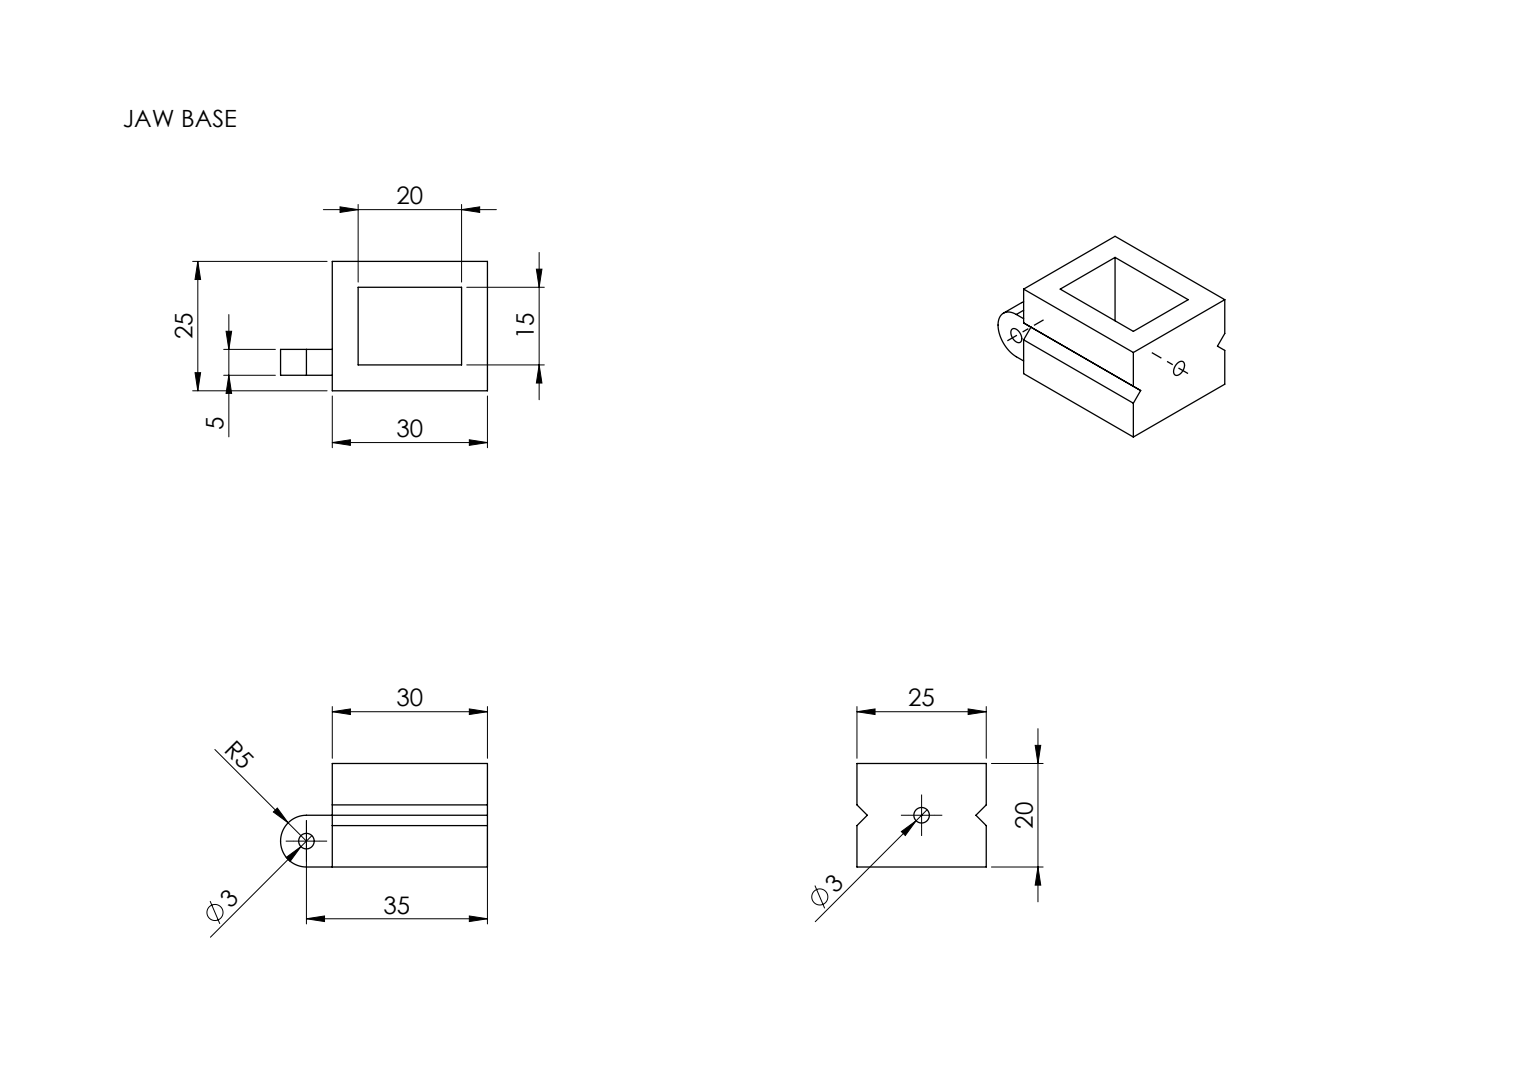
ISO-10303-21;
HEADER;
FILE_DESCRIPTION (('STEP AP214'),
    '1' );
FILE_NAME ('jaw base.step',
    '2026-10-04T07:56:41',
    ( '' ),
    ( '' ),
    'SwSTEP 2.0',
    'SolidWorks 2026',
    '' );
FILE_SCHEMA (( 'AUTOMOTIVE_DESIGN' ));
ENDSEC;

DATA;
#2=DIRECTION ( 'NONE',  ( -0.000000000000000000, 2.775557561562891351E-16, -1.000000000000000000 ) ) ;
#9=VERTEX_POINT ( 'NONE', #7435 ) ;
#11=DIRECTION ( 'NONE',  ( 0.000000000000000000, -1.000000000000000000, 0.000000000000000000 ) ) ;
#43=EDGE_CURVE ( 'NONE', #1966, #5555, #3595, .T. ) ;
#44=LINE ( 'NONE', #810, #6447 ) ;
#74=CARTESIAN_POINT ( 'NONE',  ( 54.99999999999999289, 1.301042606982605715E-15, -7.500000000000002665 ) ) ;
#76=EDGE_LOOP ( 'NONE', ( #356, #276, #5543, #6009 ) ) ;
#88=FACE_OUTER_BOUND ( 'NONE', #2763, .T. ) ;
#100=CARTESIAN_POINT ( 'NONE',  ( 50.00000000000000000, -1.734723475976807094E-15, 12.50000000000000000 ) ) ;
#116=DIRECTION ( 'NONE',  ( 0.000000000000000000, 0.000000000000000000, 1.000000000000000000 ) ) ;
#129=AXIS2_PLACEMENT_3D ( 'NONE', #1955, #4587, #1439 ) ;
#148=LINE ( 'NONE', #5288, #6329 ) ;
#154=LINE ( 'NONE', #7878, #4231 ) ;
#158=EDGE_CURVE ( 'NONE', #4876, #5889, #5061, .T. ) ;
#177=LINE ( 'NONE', #1487, #3670 ) ;
#187=VECTOR ( 'NONE', #1383, 1000.000000000000000 ) ;
#189=AXIS2_PLACEMENT_3D ( 'NONE', #3637, #5920, #5243 ) ;
#192=FACE_OUTER_BOUND ( 'NONE', #662, .T. ) ;
#210=VERTEX_POINT ( 'NONE', #510 ) ;
#226=EDGE_CURVE ( 'NONE', #6118, #4574, #2581, .T. ) ;
#266=CARTESIAN_POINT ( 'NONE',  ( 54.99999999999999289, -1.301042606982604729E-15, 7.499999999999997335 ) ) ;
#271=CIRCLE ( 'NONE', #522, 5.000000000000000888 ) ;
#276=ORIENTED_EDGE ( 'NONE', *, *, #1868, .F. ) ;
#280=EDGE_CURVE ( 'NONE', #6915, #2088, #1958, .T. ) ;
#291=ADVANCED_FACE ( 'NONE', ( #7854, #719 ), #1914, .F. ) ;
#295=CARTESIAN_POINT ( 'NONE',  ( 54.99999999999999289, 1.301042606982605715E-15, -7.500000000000002665 ) ) ;
#299=CARTESIAN_POINT ( 'NONE',  ( 50.00000000000000000, 1.734723475976807094E-15, -12.50000000000000000 ) ) ;
#305=CARTESIAN_POINT ( 'NONE',  ( 54.99999999999999289, -9.999999999999994671, -1.500000000000000666 ) ) ;
#314=CARTESIAN_POINT ( 'NONE',  ( 45.00000000000000000, -14.99999999999999467, 4.499999999999999112 ) ) ;
#328=EDGE_CURVE ( 'NONE', #3916, #5740, #1998, .T. ) ;
#344=CARTESIAN_POINT ( 'NONE',  ( 80.00000000000000000, -9.999999999999991118, -10.50000000000000888 ) ) ;
#348=VERTEX_POINT ( 'NONE', #4548 ) ;
#352=FACE_OUTER_BOUND ( 'NONE', #3772, .T. ) ;
#356=ORIENTED_EDGE ( 'NONE', *, *, #5085, .F. ) ;
#359=EDGE_CURVE ( 'NONE', #1450, #210, #2081, .T. ) ;
#373=CARTESIAN_POINT ( 'NONE',  ( 75.00000000000000000, -19.99999999999999645, -7.500000000000006217 ) ) ;
#397=AXIS2_PLACEMENT_3D ( 'NONE', #4050, #2120, #1311 ) ;
#414=EDGE_CURVE ( 'NONE', #7949, #1490, #44, .T. ) ;
#424=FACE_OUTER_BOUND ( 'NONE', #5365, .T. ) ;
#440=ORIENTED_EDGE ( 'NONE', *, *, #4555, .F. ) ;
#443=CARTESIAN_POINT ( 'NONE',  ( 50.00000000000000000, -9.999999999999994671, -1.500000000000000666 ) ) ;
#463=CARTESIAN_POINT ( 'NONE',  ( 54.99999999999999289, -19.99999999999999645, -12.50000000000000355 ) ) ;
#476=LINE ( 'NONE', #8193, #724 ) ;
#477=ADVANCED_FACE ( 'NONE', ( #88 ), #7132, .F. ) ;
#481=PLANE ( 'NONE',  #6922 ) ;
#482=ORIENTED_EDGE ( 'NONE', *, *, #2370, .T. ) ;
#499=VECTOR ( 'NONE', #7220, 1000.000000000000000 ) ;
#510=CARTESIAN_POINT ( 'NONE',  ( 50.00000000000000000, -12.00000000000000711, 12.49999999999999822 ) ) ;
#514=CARTESIAN_POINT ( 'NONE',  ( 80.00000000000000000, -7.999999999999992895, -12.50000000000000178 ) ) ;
#518=SURFACE_STYLE_USAGE ( .BOTH. , #4233 ) ;
#519=ORIENTED_EDGE ( 'NONE', *, *, #6332, .T. ) ;
#522=AXIS2_PLACEMENT_3D ( 'NONE', #3905, #2648, #1459 ) ;
#523=DIRECTION ( 'NONE',  ( 1.000000000000000000, 0.000000000000000000, 0.000000000000000000 ) ) ;
#548=PLANE ( 'NONE',  #3363 ) ;
#561=ORIENTED_EDGE ( 'NONE', *, *, #611, .F. ) ;
#562=LINE ( 'NONE', #3139, #7733 ) ;
#585=VECTOR ( 'NONE', #4039, 1000.000000000000000 ) ;
#589=AXIS2_PLACEMENT_3D ( 'NONE', #100, #733, #2054 ) ;
#611=EDGE_CURVE ( 'NONE', #5740, #6524, #3988, .T. ) ;
#618=FACE_OUTER_BOUND ( 'NONE', #620, .T. ) ;
#620=EDGE_LOOP ( 'NONE', ( #5338, #2831, #6955, #4736 ) ) ;
#637=AXIS2_PLACEMENT_3D ( 'NONE', #2916, #7427, #1567 ) ;
#641=ORIENTED_EDGE ( 'NONE', *, *, #1752, .T. ) ;
#662=EDGE_LOOP ( 'NONE', ( #2589, #4451, #6768, #2881 ) ) ;
#675=CARTESIAN_POINT ( 'NONE',  ( 50.00000000000000000, -20.00000000000000355, 12.49999999999999645 ) ) ;
#678=CARTESIAN_POINT ( 'NONE',  ( 40.00000000000000000, -9.999999999999991118, 9.499999999999998224 ) ) ;
#694=EDGE_CURVE ( 'NONE', #3832, #7792, #3206, .T. ) ;
#700=AXIS2_PLACEMENT_3D ( 'NONE', #5107, #2634, #5148 ) ;
#703=DIRECTION ( 'NONE',  ( -1.000000000000000000, -0.000000000000000000, -0.000000000000000000 ) ) ;
#719=FACE_OUTER_BOUND ( 'NONE', #1634, .T. ) ;
#722=FACE_BOUND ( 'NONE', #2870, .T. ) ;
#724=VECTOR ( 'NONE', #4868, 1000.000000000000114 ) ;
#733=DIRECTION ( 'NONE',  ( 0.000000000000000000, -2.168404344971010347E-16, 1.000000000000000000 ) ) ;
#734=EDGE_CURVE ( 'NONE', #4784, #5781, #271, .T. ) ;
#740=DIRECTION ( 'NONE',  ( 0.000000000000000000, 0.000000000000000000, -1.000000000000000000 ) ) ;
#748=LINE ( 'NONE', #5933, #187 ) ;
#758=CARTESIAN_POINT ( 'NONE',  ( 45.00000000000000000, -15.00000000000000000, -4.163336342344337027E-15 ) ) ;
#778=DIRECTION ( 'NONE',  ( -0.000000000000000000, 1.000000000000000000, 1.734723475976807094E-16 ) ) ;
#781=DIRECTION ( 'NONE',  ( -0.000000000000000000, -1.387778780781445676E-16, 1.000000000000000000 ) ) ;
#784=DIRECTION ( 'NONE',  ( 1.000000000000000000, 0.000000000000000000, 0.000000000000000000 ) ) ;
#789=ORIENTED_EDGE ( 'NONE', *, *, #1868, .T. ) ;
#791=LINE ( 'NONE', #5465, #585 ) ;
#802=VECTOR ( 'NONE', #5944, 1000.000000000000000 ) ;
#810=CARTESIAN_POINT ( 'NONE',  ( 50.00000000000000000, -19.99999999999999645, -12.50000000000000355 ) ) ;
#832=ORIENTED_EDGE ( 'NONE', *, *, #1520, .T. ) ;
#842=EDGE_CURVE ( 'NONE', #7792, #3832, #1325, .T. ) ;
#845=FACE_OUTER_BOUND ( 'NONE', #4405, .T. ) ;
#852=CYLINDRICAL_SURFACE ( 'NONE', #6905, 1.500000000000000666 ) ;
#858=ORIENTED_EDGE ( 'NONE', *, *, #2230, .T. ) ;
#867=DIRECTION ( 'NONE',  ( 0.000000000000000000, -1.000000000000000000, 3.469446951953615175E-16 ) ) ;
#871=CARTESIAN_POINT ( 'NONE',  ( 50.00000000000000000, -9.999999999999992895, 4.499999999999999112 ) ) ;
#876=CARTESIAN_POINT ( 'NONE',  ( 50.00000000000000000, -12.00000000000000355, -12.50000000000000178 ) ) ;
#879=ADVANCED_FACE ( 'NONE', ( #1961 ), #7726, .F. ) ;
#889=FACE_BOUND ( 'NONE', #8067, .T. ) ;
#893=CARTESIAN_POINT ( 'NONE',  ( 50.00000000000000000, -9.999999999999994671, 10.50000000000000533 ) ) ;
#903=EDGE_CURVE ( 'NONE', #1902, #2390, #2584, .T. ) ;
#914=VERTEX_POINT ( 'NONE', #3261 ) ;
#918=ORIENTED_EDGE ( 'NONE', *, *, #4017, .T. ) ;
#957=PLANE ( 'NONE',  #3547 ) ;
#960=ADVANCED_FACE ( 'NONE', ( #722, #3931 ), #2758, .F. ) ;
#968=EDGE_LOOP ( 'NONE', ( #6723, #4873, #5987, #7324 ) ) ;
#992=APPLICATION_CONTEXT ( 'automotive_design' ) ;
#1003=ORIENTED_EDGE ( 'NONE', *, *, #842, .F. ) ;
#1013=DIRECTION ( 'NONE',  ( 0.000000000000000000, 0.7071067811865442421, -0.7071067811865509034 ) ) ;
#1022=DIRECTION ( 'NONE',  ( 0.000000000000000000, 0.000000000000000000, -1.000000000000000000 ) ) ;
#1040=EDGE_LOOP ( 'NONE', ( #1925, #1101, #1165, #6177 ) ) ;
#1060=EDGE_CURVE ( 'NONE', #6118, #5503, #2083, .T. ) ;
#1063=CYLINDRICAL_SURFACE ( 'NONE', #189, 1.500000000000000666 ) ;
#1072=MECHANICAL_DESIGN_GEOMETRIC_PRESENTATION_REPRESENTATION('',(#7261),#2289);
#1081=LINE ( 'NONE', #4358, #6236 ) ;
#1101=ORIENTED_EDGE ( 'NONE', *, *, #5827, .T. ) ;
#1116=ORIENTED_EDGE ( 'NONE', *, *, #8084, .T. ) ;
#1119=ORIENTED_EDGE ( 'NONE', *, *, #4522, .F. ) ;
#1122=VECTOR ( 'NONE', #1414, 1000.000000000000000 ) ;
#1133=VECTOR ( 'NONE', #778, 1000.000000000000000 ) ;
#1135=PRODUCT_DEFINITION ( 'UNKNOWN', '', #8199, #8065 ) ;
#1159=ADVANCED_FACE ( 'NONE', ( #6622 ), #6113, .F. ) ;
#1163=DIRECTION ( 'NONE',  ( 0.000000000000000000, 2.775557561562891351E-16, -1.000000000000000000 ) ) ;
#1165=ORIENTED_EDGE ( 'NONE', *, *, #4237, .T. ) ;
#1166=DIRECTION ( 'NONE',  ( 1.000000000000000000, -0.000000000000000000, -0.000000000000000000 ) ) ;
#1176=ORIENTED_EDGE ( 'NONE', *, *, #6774, .T. ) ;
#1192=CARTESIAN_POINT ( 'NONE',  ( 50.00000000000000000, -12.00000000000000355, -12.50000000000000178 ) ) ;
#1200=ORIENTED_EDGE ( 'NONE', *, *, #6332, .F. ) ;
#1203=CARTESIAN_POINT ( 'NONE',  ( 45.00000000000000000, -19.99999999999999645, -12.50000000000000355 ) ) ;
#1207=ORIENTED_EDGE ( 'NONE', *, *, #4767, .T. ) ;
#1229=EDGE_CURVE ( 'NONE', #4621, #6524, #2166, .T. ) ;
#1244=ORIENTED_EDGE ( 'NONE', *, *, #6774, .F. ) ;
#1258=CARTESIAN_POINT ( 'NONE',  ( 75.00000000000000000, -30.00000000000000000, -7.500000000000007105 ) ) ;
#1289=EDGE_CURVE ( 'NONE', #5070, #3705, #5351, .T. ) ;
#1294=CARTESIAN_POINT ( 'NONE',  ( 46.49999999999999289, -14.99999999999999467, 9.499999999999996447 ) ) ;
#1299=CARTESIAN_POINT ( 'NONE',  ( 80.00000000000000000, 1.734723475976807094E-15, -12.50000000000000000 ) ) ;
#1302=ORIENTED_EDGE ( 'NONE', *, *, #3633, .T. ) ;
#1311=DIRECTION ( 'NONE',  ( 0.000000000000000000, -1.000000000000000000, 8.673617379884033007E-17 ) ) ;
#1317=DIRECTION ( 'NONE',  ( -0.000000000000000000, 0.7071067811865484609, -0.7071067811865465735 ) ) ;
#1320=EDGE_CURVE ( 'NONE', #9, #5499, #4213, .T. ) ;
#1325=CIRCLE ( 'NONE', #4616, 1.500000000000000666 ) ;
#1328=VECTOR ( 'NONE', #5772, 1000.000000000000000 ) ;
#1348=AXIS2_PLACEMENT_3D ( 'NONE', #6049, #867, #2180 ) ;
#1353=MECHANICAL_DESIGN_GEOMETRIC_PRESENTATION_REPRESENTATION('',(#7140),#3380);
#1375=DIRECTION ( 'NONE',  ( -1.000000000000000000, -0.000000000000000000, -0.000000000000000000 ) ) ;
#1383=DIRECTION ( 'NONE',  ( -0.000000000000000000, 2.775557561562891351E-16, -1.000000000000000000 ) ) ;
#1393=LINE ( 'NONE', #3386, #802 ) ;
#1414=DIRECTION ( 'NONE',  ( -0.000000000000000000, -3.469446951953614682E-16, -1.000000000000000000 ) ) ;
#1419=DIRECTION ( 'NONE',  ( -1.000000000000000000, -0.000000000000000000, -0.000000000000000000 ) ) ;
#1421=APPLICATION_CONTEXT ( 'automotive_design' ) ;
#1439=DIRECTION ( 'NONE',  ( 0.000000000000000000, 0.000000000000000000, -1.000000000000000000 ) ) ;
#1445=LINE ( 'NONE', #2167, #3270 ) ;
#1450=VERTEX_POINT ( 'NONE', #893 ) ;
#1451=VECTOR ( 'NONE', #6786, 1000.000000000000000 ) ;
#1459=DIRECTION ( 'NONE',  ( 0.000000000000000000, 1.000000000000000000, 0.000000000000000000 ) ) ;
#1464=ADVANCED_FACE ( 'NONE', ( #7342 ), #4174, .T. ) ;
#1481=AXIS2_PLACEMENT_3D ( 'NONE', #6071, #6783, #2872 ) ;
#1487=CARTESIAN_POINT ( 'NONE',  ( 80.00000000000000000, -1.734723475976807094E-15, 12.50000000000000000 ) ) ;
#1490=VERTEX_POINT ( 'NONE', #5600 ) ;
#1499=LINE ( 'NONE', #1630, #2833 ) ;
#1507=ORIENTED_EDGE ( 'NONE', *, *, #1229, .T. ) ;
#1508=CARTESIAN_POINT ( 'NONE',  ( 80.00000000000000000, -12.00000000000000355, -12.50000000000000178 ) ) ;
#1511=ORIENTED_EDGE ( 'NONE', *, *, #6199, .T. ) ;
#1520=EDGE_CURVE ( 'NONE', #5848, #6118, #2330, .T. ) ;
#1526=DIRECTION ( 'NONE',  ( -0.000000000000000000, -8.673617379884033007E-17, -1.000000000000000000 ) ) ;
#1538=AXIS2_PLACEMENT_3D ( 'NONE', #2727, #3719, #7552 ) ;
#1539=AXIS2_PLACEMENT_3D ( 'NONE', #6210, #4308, #8076 ) ;
#1544=EDGE_LOOP ( 'NONE', ( #2817, #1646, #7710, #7360 ) ) ;
#1549=CLOSED_SHELL ( 'NONE', ( #879, #7015, #477, #7270, #2468, #1870, #1464, #4583, #5249, #6031, #2053, #5963, #7130, #6092, #5785, #960, #4435, #7621, #3038, #8204, #1159, #291, #8313, #7524, #5577, #7294, #6000 ) ) ;
#1563=DIRECTION ( 'NONE',  ( 0.000000000000000000, -1.734723475976807094E-16, 1.000000000000000000 ) ) ;
#1567=DIRECTION ( 'NONE',  ( 0.000000000000000000, 1.000000000000000000, 1.734723475976807094E-16 ) ) ;
#1574=CARTESIAN_POINT ( 'NONE',  ( 43.50000000000000711, -14.99999999999999467, 4.499999999999999112 ) ) ;
#1581=DIRECTION ( 'NONE',  ( 1.000000000000000000, 0.000000000000000000, 0.000000000000000000 ) ) ;
#1601=VECTOR ( 'NONE', #2366, 1000.000000000000000 ) ;
#1603=FACE_OUTER_BOUND ( 'NONE', #4496, .T. ) ;
#1604=VECTOR ( 'NONE', #3130, 1000.000000000000000 ) ;
#1612=DIRECTION ( 'NONE',  ( 0.000000000000000000, -1.000000000000000000, -2.168404344971010347E-16 ) ) ;
#1614=DIRECTION ( 'NONE',  ( -0.000000000000000000, -0.000000000000000000, 1.000000000000000000 ) ) ;
#1630=CARTESIAN_POINT ( 'NONE',  ( 50.00000000000000000, -9.999999999999991118, -10.50000000000000888 ) ) ;
#1632=EDGE_LOOP ( 'NONE', ( #7359, #4290, #4858, #4408, #7822, #4478, #3099, #1119, #7706, #6680, #5713, #6083, #5517, #2025 ) ) ;
#1634=EDGE_LOOP ( 'NONE', ( #8213, #7096, #1511, #918, #7592 ) ) ;
#1646=ORIENTED_EDGE ( 'NONE', *, *, #7805, .F. ) ;
#1647=CARTESIAN_POINT ( 'NONE',  ( 45.00000000000000000, -19.99999999999999645, 4.500000000000000000 ) ) ;
#1658=VERTEX_POINT ( 'NONE', #1294 ) ;
#1660=CARTESIAN_POINT ( 'NONE',  ( 50.00000000000000000, -9.999999999999994671, 1.500000000000000666 ) ) ;
#1670=SURFACE_STYLE_FILL_AREA ( #2933 ) ;
#1673=VERTEX_POINT ( 'NONE', #4445 ) ;
#1701=LINE ( 'NONE', #3757, #1884 ) ;
#1703=DIRECTION ( 'NONE',  ( -0.000000000000000000, -0.000000000000000000, 1.000000000000000000 ) ) ;
#1710=CARTESIAN_POINT ( 'NONE',  ( 54.99999999999999289, -30.00000000000000000, -7.500000000000007105 ) ) ;
#1712=( NAMED_UNIT ( * ) SI_UNIT ( $, .STERADIAN. ) SOLID_ANGLE_UNIT ( ) );
#1715=CARTESIAN_POINT ( 'NONE',  ( 75.00000000000000000, -19.99999999999999645, -12.50000000000000355 ) ) ;
#1716=PRODUCT ( 'jaw base', 'jaw base', '', ( #5739 ) ) ;
#1717=ORIENTED_EDGE ( 'NONE', *, *, #5266, .F. ) ;
#1732=LINE ( 'NONE', #8253, #1601 ) ;
#1740=( LENGTH_UNIT ( ) NAMED_UNIT ( * ) SI_UNIT ( .MILLI., .METRE. ) );
#1741=ORIENTED_EDGE ( 'NONE', *, *, #7805, .T. ) ;
#1744=VECTOR ( 'NONE', #5258, 1000.000000000000000 ) ;
#1750=DIRECTION ( 'NONE',  ( 1.000000000000000000, -0.000000000000000000, -0.000000000000000000 ) ) ;
#1752=EDGE_CURVE ( 'NONE', #3497, #6231, #2813, .T. ) ;
#1756=DIRECTION ( 'NONE',  ( 1.000000000000000000, 0.000000000000000000, 0.000000000000000000 ) ) ;
#1793=EDGE_CURVE ( 'NONE', #5848, #1966, #154, .T. ) ;
#1797=( LENGTH_UNIT ( ) NAMED_UNIT ( * ) SI_UNIT ( .MILLI., .METRE. ) );
#1804=AXIS2_PLACEMENT_3D ( 'NONE', #5339, #7884, #7325 ) ;
#1812=VECTOR ( 'NONE', #4475, 1000.000000000000000 ) ;
#1819=VERTEX_POINT ( 'NONE', #871 ) ;
#1827=ORIENTED_EDGE ( 'NONE', *, *, #6199, .F. ) ;
#1838=LINE ( 'NONE', #4470, #1924 ) ;
#1857=DIRECTION ( 'NONE',  ( 1.000000000000000000, 0.000000000000000000, 0.000000000000000000 ) ) ;
#1860=ORIENTED_EDGE ( 'NONE', *, *, #3440, .F. ) ;
#1868=EDGE_CURVE ( 'NONE', #210, #8159, #4313, .T. ) ;
#1870=ADVANCED_FACE ( 'NONE', ( #2353, #3017 ), #481, .T. ) ;
#1884=VECTOR ( 'NONE', #8224, 1000.000000000000000 ) ;
#1901=CARTESIAN_POINT ( 'NONE',  ( 50.00000000000000000, -7.999999999999992895, -12.50000000000000178 ) ) ;
#1902=VERTEX_POINT ( 'NONE', #6846 ) ;
#1910=DIRECTION ( 'NONE',  ( -0.000000000000000000, 0.7071067811865442421, 0.7071067811865509034 ) ) ;
#1914=PLANE ( 'NONE',  #6045 ) ;
#1918=LINE ( 'NONE', #514, #2199 ) ;
#1919=EDGE_CURVE ( 'NONE', #5503, #914, #7407, .T. ) ;
#1924=VECTOR ( 'NONE', #8233, 1000.000000000000000 ) ;
#1925=ORIENTED_EDGE ( 'NONE', *, *, #1060, .T. ) ;
#1955=CARTESIAN_POINT ( 'NONE',  ( 50.00000000000000000, -9.999999999999994671, 0.000000000000000000 ) ) ;
#1958=LINE ( 'NONE', #4465, #4286 ) ;
#1961=FACE_OUTER_BOUND ( 'NONE', #7933, .T. ) ;
#1966=VERTEX_POINT ( 'NONE', #6133 ) ;
#1982=ORIENTED_EDGE ( 'NONE', *, *, #7035, .T. ) ;
#1998=LINE ( 'NONE', #6413, #1328 ) ;
#2001=CARTESIAN_POINT ( 'NONE',  ( 45.00000000000000000, -14.99999999999999467, -12.50000000000000178 ) ) ;
#2002=DIRECTION ( 'NONE',  ( 1.000000000000000000, 0.000000000000000000, 0.000000000000000000 ) ) ;
#2006=ORIENTED_EDGE ( 'NONE', *, *, #158, .F. ) ;
#2025=ORIENTED_EDGE ( 'NONE', *, *, #6810, .F. ) ;
#2026=CARTESIAN_POINT ( 'NONE',  ( 45.00000000000000000, -19.99999999999999645, 9.500000000000000000 ) ) ;
#2039=FACE_OUTER_BOUND ( 'NONE', #6713, .T. ) ;
#2053=ADVANCED_FACE ( 'NONE', ( #3691, #4355 ), #6262, .T. ) ;
#2054=DIRECTION ( 'NONE',  ( 0.000000000000000000, -1.000000000000000000, -2.168404344971010347E-16 ) ) ;
#2055=LINE ( 'NONE', #4603, #1133 ) ;
#2066=DIRECTION ( 'NONE',  ( 0.000000000000000000, -1.000000000000000000, 3.469446951953616161E-16 ) ) ;
#2080=VECTOR ( 'NONE', #1703, 1000.000000000000000 ) ;
#2081=LINE ( 'NONE', #5814, #3620 ) ;
#2083=LINE ( 'NONE', #4638, #499 ) ;
#2088=VERTEX_POINT ( 'NONE', #6805 ) ;
#2091=AXIS2_PLACEMENT_3D ( 'NONE', #3056, #4236, #1163 ) ;
#2092=EDGE_CURVE ( 'NONE', #9, #1819, #8198, .T. ) ;
#2107=ORIENTED_EDGE ( 'NONE', *, *, #3963, .F. ) ;
#2120=DIRECTION ( 'NONE',  ( 0.000000000000000000, 8.673617379884033007E-17, 1.000000000000000000 ) ) ;
#2139=DIRECTION ( 'NONE',  ( -0.000000000000000000, 0.7071067811865507924, 0.7071067811865441310 ) ) ;
#2143=CARTESIAN_POINT ( 'NONE',  ( 50.00000000000000000, -19.99999999999999645, -12.50000000000000355 ) ) ;
#2150=DIRECTION ( 'NONE',  ( 0.000000000000000000, -0.7071067811865485719, -0.7071067811865465735 ) ) ;
#2161=LINE ( 'NONE', #5394, #8070 ) ;
#2166=LINE ( 'NONE', #5482, #6827 ) ;
#2167=CARTESIAN_POINT ( 'NONE',  ( 40.00000000000000000, -9.999999999999991118, 9.499999999999998224 ) ) ;
#2180=DIRECTION ( 'NONE',  ( 0.000000000000000000, -3.469446951953615175E-16, -1.000000000000000000 ) ) ;
#2183=ORIENTED_EDGE ( 'NONE', *, *, #226, .T. ) ;
#2190=LINE ( 'NONE', #74, #6378 ) ;
#2199=VECTOR ( 'NONE', #5732, 1000.000000000000000 ) ;
#2230=EDGE_CURVE ( 'NONE', #5781, #5070, #3898, .T. ) ;
#2232=CARTESIAN_POINT ( 'NONE',  ( 54.99999999999999289, -19.99999999999999645, -7.500000000000006217 ) ) ;
#2259=VERTEX_POINT ( 'NONE', #3268 ) ;
#2268=ORIENTED_EDGE ( 'NONE', *, *, #5676, .T. ) ;
#2285=LINE ( 'NONE', #295, #2295 ) ;
#2289=( GEOMETRIC_REPRESENTATION_CONTEXT ( 3 ) GLOBAL_UNCERTAINTY_ASSIGNED_CONTEXT ( ( #5541 ) ) GLOBAL_UNIT_ASSIGNED_CONTEXT ( ( #1740, #4299, #3082 ) ) REPRESENTATION_CONTEXT ( 'NONE', 'WORKASPACE' ) );
#2295=VECTOR ( 'NONE', #1563, 1000.000000000000000 ) ;
#2302=EDGE_LOOP ( 'NONE', ( #1741, #7262 ) ) ;
#2330=LINE ( 'NONE', #463, #5485 ) ;
#2342=DIRECTION ( 'NONE',  ( 0.000000000000000000, -1.000000000000000000, -2.168404344971009854E-16 ) ) ;
#2344=EDGE_CURVE ( 'NONE', #4647, #6779, #3826, .T. ) ;
#2353=FACE_BOUND ( 'NONE', #7797, .T. ) ;
#2356=DIRECTION ( 'NONE',  ( 1.000000000000000000, 0.000000000000000000, 0.000000000000000000 ) ) ;
#2365=ORIENTED_EDGE ( 'NONE', *, *, #5011, .F. ) ;
#2366=DIRECTION ( 'NONE',  ( 0.000000000000000000, -1.000000000000000000, 8.673617379884034239E-17 ) ) ;
#2370=EDGE_CURVE ( 'NONE', #3916, #4621, #562, .T. ) ;
#2390=VERTEX_POINT ( 'NONE', #4432 ) ;
#2405=EDGE_LOOP ( 'NONE', ( #4179, #3289, #4917, #1860 ) ) ;
#2430=CARTESIAN_POINT ( 'NONE',  ( 40.00000000000000000, -9.999999999999992895, 4.499999999999999112 ) ) ;
#2468=ADVANCED_FACE ( 'NONE', ( #6044 ), #2768, .T. ) ;
#2473=LINE ( 'NONE', #4277, #4084 ) ;
#2486=ORIENTED_EDGE ( 'NONE', *, *, #8250, .T. ) ;
#2489=ORIENTED_EDGE ( 'NONE', *, *, #4223, .T. ) ;
#2504=CARTESIAN_POINT ( 'NONE',  ( 80.00000000000000000, -9.999999999999994671, 0.000000000000000000 ) ) ;
#2523=CARTESIAN_POINT ( 'NONE',  ( 54.99999999999999289, -20.00000000000000000, 7.499999999999993783 ) ) ;
#2524=LINE ( 'NONE', #5088, #4898 ) ;
#2529=VECTOR ( 'NONE', #1317, 1000.000000000000000 ) ;
#2539=DIRECTION ( 'NONE',  ( 0.000000000000000000, 0.000000000000000000, -1.000000000000000000 ) ) ;
#2550=VECTOR ( 'NONE', #3673, 1000.000000000000000 ) ;
#2552=SHAPE_DEFINITION_REPRESENTATION ( #8309, #6502 ) ;
#2564=DIRECTION ( 'NONE',  ( 0.000000000000000000, 2.775557561562891351E-16, -1.000000000000000000 ) ) ;
#2578=CARTESIAN_POINT ( 'NONE',  ( 50.00000000000000000, -9.999999999999991118, 9.499999999999998224 ) ) ;
#2581=LINE ( 'NONE', #2630, #3756 ) ;
#2584=LINE ( 'NONE', #5904, #2529 ) ;
#2589=ORIENTED_EDGE ( 'NONE', *, *, #5149, .T. ) ;
#2611=CARTESIAN_POINT ( 'NONE',  ( 50.00000000000000000, -1.734723475976807094E-15, 12.50000000000000000 ) ) ;
#2617=VECTOR ( 'NONE', #1750, 1000.000000000000000 ) ;
#2624=VECTOR ( 'NONE', #6763, 1000.000000000000000 ) ;
#2630=CARTESIAN_POINT ( 'NONE',  ( 54.99999999999999289, -30.00000000000000000, -7.500000000000007105 ) ) ;
#2634=DIRECTION ( 'NONE',  ( 0.000000000000000000, 1.734723475976806108E-16, 1.000000000000000000 ) ) ;
#2648=DIRECTION ( 'NONE',  ( 0.000000000000000000, 1.734723475976806108E-16, 1.000000000000000000 ) ) ;
#2671=CARTESIAN_POINT ( 'NONE',  ( 50.00000000000000000, -9.999999999999994671, 0.000000000000000000 ) ) ;
#2675=CARTESIAN_POINT ( 'NONE',  ( 80.00000000000000000, 0.000000000000000000, 0.000000000000000000 ) ) ;
#2688=LINE ( 'NONE', #5874, #6857 ) ;
#2690=VECTOR ( 'NONE', #4504, 1000.000000000000000 ) ;
#2727=CARTESIAN_POINT ( 'NONE',  ( 54.99999999999999289, -9.999999999999994671, 0.000000000000000000 ) ) ;
#2733=DIRECTION ( 'NONE',  ( 0.000000000000000000, 0.000000000000000000, -1.000000000000000000 ) ) ;
#2743=ORIENTED_EDGE ( 'NONE', *, *, #734, .F. ) ;
#2751=FACE_BOUND ( 'NONE', #7838, .T. ) ;
#2758=PLANE ( 'NONE',  #8053 ) ;
#2759=CARTESIAN_POINT ( 'NONE',  ( 50.00000000000000000, -20.00000000000000000, 4.499999999999997335 ) ) ;
#2762=AXIS2_PLACEMENT_3D ( 'NONE', #7398, #4187, #3558 ) ;
#2763=EDGE_LOOP ( 'NONE', ( #6738, #2922, #3529, #440 ) ) ;
#2768=PLANE ( 'NONE',  #589 ) ;
#2771=PLANE ( 'NONE',  #8210 ) ;
#2779=VERTEX_POINT ( 'NONE', #4911 ) ;
#2780=CARTESIAN_POINT ( 'NONE',  ( 50.00000000000000000, -7.999999999999996447, 12.49999999999999822 ) ) ;
#2789=EDGE_CURVE ( 'NONE', #3705, #9, #3018, .T. ) ;
#2813=LINE ( 'NONE', #2143, #6116 ) ;
#2817=ORIENTED_EDGE ( 'NONE', *, *, #280, .F. ) ;
#2831=ORIENTED_EDGE ( 'NONE', *, *, #2789, .F. ) ;
#2833=VECTOR ( 'NONE', #2139, 1000.000000000000114 ) ;
#2840=AXIS2_PLACEMENT_3D ( 'NONE', #8120, #5497, #1756 ) ;
#2852=DIRECTION ( 'NONE',  ( 0.000000000000000000, -1.734723475976807094E-16, 1.000000000000000000 ) ) ;
#2855=VERTEX_POINT ( 'NONE', #5614 ) ;
#2870=EDGE_LOOP ( 'NONE', ( #3399, #1717 ) ) ;
#2872=DIRECTION ( 'NONE',  ( 0.000000000000000000, 0.000000000000000000, -1.000000000000000000 ) ) ;
#2876=DIRECTION ( 'NONE',  ( 0.000000000000000000, 2.168404344971010347E-16, -1.000000000000000000 ) ) ;
#2881=ORIENTED_EDGE ( 'NONE', *, *, #7035, .F. ) ;
#2894=CARTESIAN_POINT ( 'NONE',  ( 54.99999999999999289, -30.00000000000000000, 7.499999999999992006 ) ) ;
#2898=EDGE_CURVE ( 'NONE', #5070, #3497, #4230, .T. ) ;
#2912=DIRECTION ( 'NONE',  ( 1.000000000000000000, 0.000000000000000000, 0.000000000000000000 ) ) ;
#2916=CARTESIAN_POINT ( 'NONE',  ( 54.99999999999999289, -30.00000000000000000, -7.500000000000007105 ) ) ;
#2922=ORIENTED_EDGE ( 'NONE', *, *, #3935, .T. ) ;
#2933=FILL_AREA_STYLE ('',( #7443 ) ) ;
#2947=VECTOR ( 'NONE', #8056, 1000.000000000000000 ) ;
#2970=PLANE ( 'NONE',  #4352 ) ;
#2972=( LENGTH_UNIT ( ) NAMED_UNIT ( * ) SI_UNIT ( .MILLI., .METRE. ) );
#2974=VERTEX_POINT ( 'NONE', #6758 ) ;
#2976=EDGE_CURVE ( 'NONE', #2259, #1658, #5695, .T. ) ;
#2978=LINE ( 'NONE', #6850, #3812 ) ;
#2995=VECTOR ( 'NONE', #2002, 1000.000000000000000 ) ;
#2998=SURFACE_STYLE_USAGE ( .BOTH. , #6913 ) ;
#2999=EDGE_LOOP ( 'NONE', ( #7017, #1200, #3245, #3998 ) ) ;
#3004=EDGE_CURVE ( 'NONE', #210, #7949, #3052, .T. ) ;
#3017=FACE_OUTER_BOUND ( 'NONE', #6625, .T. ) ;
#3018=CIRCLE ( 'NONE', #1539, 5.000000000000000888 ) ;
#3038=ADVANCED_FACE ( 'NONE', ( #352, #5495 ), #2970, .F. ) ;
#3043=EDGE_CURVE ( 'NONE', #2779, #8159, #476, .T. ) ;
#3052=LINE ( 'NONE', #6127, #7320 ) ;
#3056=CARTESIAN_POINT ( 'NONE',  ( 50.00000000000000000, -19.99999999999999645, -12.50000000000000355 ) ) ;
#3082=( NAMED_UNIT ( * ) SI_UNIT ( $, .STERADIAN. ) SOLID_ANGLE_UNIT ( ) );
#3083=ORIENTED_EDGE ( 'NONE', *, *, #2344, .T. ) ;
#3095=ADVANCED_BREP_SHAPE_REPRESENTATION ( '', ( #4543, #2840 ), #7820 ) ;
#3099=ORIENTED_EDGE ( 'NONE', *, *, #8084, .F. ) ;
#3100=EDGE_CURVE ( 'NONE', #6915, #6387, #4228, .T. ) ;
#3116=CARTESIAN_POINT ( 'NONE',  ( 45.00000000000000000, -9.999999999999991118, 9.499999999999998224 ) ) ;
#3130=DIRECTION ( 'NONE',  ( 1.000000000000000000, 0.000000000000000000, 0.000000000000000000 ) ) ;
#3139=CARTESIAN_POINT ( 'NONE',  ( 50.00000000000000000, -1.734723475976807094E-15, 12.50000000000000000 ) ) ;
#3143=VECTOR ( 'NONE', #6320, 1000.000000000000000 ) ;
#3159=CARTESIAN_POINT ( 'NONE',  ( 50.00000000000000000, 0.000000000000000000, 0.000000000000000000 ) ) ;
#3169=CARTESIAN_POINT ( 'NONE',  ( 46.49999999999999289, -14.99999999999999467, 4.499999999999999112 ) ) ;
#3178=EDGE_CURVE ( 'NONE', #5499, #4784, #5829, .T. ) ;
#3182=SHAPE_REPRESENTATION_RELATIONSHIP ( 'NONE' , 'NONE' ,  #6502, #3095 ) ;
#3198=ORIENTED_EDGE ( 'NONE', *, *, #2344, .F. ) ;
#3199=LINE ( 'NONE', #1299, #1744 ) ;
#3200=DIRECTION ( 'NONE',  ( 1.000000000000000000, 0.000000000000000000, -0.000000000000000000 ) ) ;
#3206=CIRCLE ( 'NONE', #7922, 1.500000000000000666 ) ;
#3210=CARTESIAN_POINT ( 'NONE',  ( 40.00000000000000000, -14.99999999999999112, 9.499999999999998224 ) ) ;
#3224=ORIENTED_EDGE ( 'NONE', *, *, #43, .F. ) ;
#3240=EDGE_CURVE ( 'NONE', #6843, #4159, #1918, .T. ) ;
#3243=LINE ( 'NONE', #1901, #7996 ) ;
#3245=ORIENTED_EDGE ( 'NONE', *, *, #6870, .T. ) ;
#3253=EDGE_CURVE ( 'NONE', #1902, #6843, #1838, .T. ) ;
#3255=DIRECTION ( 'NONE',  ( 0.000000000000000000, -1.000000000000000000, -2.775557561562891844E-16 ) ) ;
#3261=CARTESIAN_POINT ( 'NONE',  ( 75.00000000000000000, -20.00000000000000355, 7.499999999999993783 ) ) ;
#3268=CARTESIAN_POINT ( 'NONE',  ( 43.50000000000000711, -14.99999999999999467, 9.499999999999996447 ) ) ;
#3270=VECTOR ( 'NONE', #6665, 1000.000000000000000 ) ;
#3289=ORIENTED_EDGE ( 'NONE', *, *, #280, .T. ) ;
#3299=CARTESIAN_POINT ( 'NONE',  ( 50.00000000000000000, -12.00000000000000355, -12.50000000000000178 ) ) ;
#3303=DIRECTION ( 'NONE',  ( 1.000000000000000000, 0.000000000000000000, 0.000000000000000000 ) ) ;
#3328=DIRECTION ( 'NONE',  ( -1.000000000000000000, -0.000000000000000000, 0.000000000000000000 ) ) ;
#3331=ORIENTED_EDGE ( 'NONE', *, *, #7782, .F. ) ;
#3340=LINE ( 'NONE', #675, #7950 ) ;
#3346=DIRECTION ( 'NONE',  ( -0.000000000000000000, -1.387778780781445676E-16, 1.000000000000000000 ) ) ;
#3356=EDGE_CURVE ( 'NONE', #2974, #348, #5143, .T. ) ;
#3357=FACE_OUTER_BOUND ( 'NONE', #2405, .T. ) ;
#3361=DIRECTION ( 'NONE',  ( 0.000000000000000000, 8.673617379884033007E-17, 1.000000000000000000 ) ) ;
#3363=AXIS2_PLACEMENT_3D ( 'NONE', #5603, #7472, #7591 ) ;
#3373=DIRECTION ( 'NONE',  ( 0.000000000000000000, -1.000000000000000000, -2.168404344971010101E-16 ) ) ;
#3380=( GEOMETRIC_REPRESENTATION_CONTEXT ( 3 ) GLOBAL_UNCERTAINTY_ASSIGNED_CONTEXT ( ( #7302 ) ) GLOBAL_UNIT_ASSIGNED_CONTEXT ( ( #2972, #4989, #7775 ) ) REPRESENTATION_CONTEXT ( 'NONE', 'WORKASPACE' ) );
#3386=CARTESIAN_POINT ( 'NONE',  ( 40.00000000000000000, -14.99999999999999289, 4.500000000000000888 ) ) ;
#3399=ORIENTED_EDGE ( 'NONE', *, *, #3356, .F. ) ;
#3413=FACE_OUTER_BOUND ( 'NONE', #4437, .T. ) ;
#3433=UNCERTAINTY_MEASURE_WITH_UNIT (LENGTH_MEASURE( 1.000000000000000082E-05 ), #1797, 'distance_accuracy_value', 'NONE');
#3434=CARTESIAN_POINT ( 'NONE',  ( 50.00000000000000000, -9.999999999999994671, 0.000000000000000000 ) ) ;
#3438=ORIENTED_EDGE ( 'NONE', *, *, #4555, .T. ) ;
#3440=EDGE_CURVE ( 'NONE', #6387, #6901, #4720, .T. ) ;
#3454=ORIENTED_EDGE ( 'NONE', *, *, #3661, .T. ) ;
#3486=CIRCLE ( 'NONE', #6845, 1.500000000000000666 ) ;
#3497=VERTEX_POINT ( 'NONE', #2759 ) ;
#3501=CARTESIAN_POINT ( 'NONE',  ( 75.00000000000000000, -9.999999999999994671, 1.500000000000000666 ) ) ;
#3512=CARTESIAN_POINT ( 'NONE',  ( 80.00000000000000000, -20.00000000000000355, 12.49999999999999645 ) ) ;
#3519=CARTESIAN_POINT ( 'NONE',  ( 40.00000000000000000, -19.99999999999999645, 4.500000000000000000 ) ) ;
#3526=CARTESIAN_POINT ( 'NONE',  ( 50.00000000000000000, -12.00000000000000711, 12.49999999999999822 ) ) ;
#3529=ORIENTED_EDGE ( 'NONE', *, *, #5266, .T. ) ;
#3535=EDGE_CURVE ( 'NONE', #5499, #7328, #1445, .T. ) ;
#3543=CARTESIAN_POINT ( 'NONE',  ( 45.00000000000000000, -15.00000000000000178, 4.500000000000000000 ) ) ;
#3547=AXIS2_PLACEMENT_3D ( 'NONE', #3526, #5301, #3373 ) ;
#3556=AXIS2_PLACEMENT_3D ( 'NONE', #7519, #1581, #6461 ) ;
#3558=DIRECTION ( 'NONE',  ( 1.000000000000000000, 0.000000000000000000, 0.000000000000000000 ) ) ;
#3580=DIRECTION ( 'NONE',  ( 0.000000000000000000, 0.000000000000000000, 1.000000000000000000 ) ) ;
#3586=CARTESIAN_POINT ( 'NONE',  ( 45.00000000000000000, -9.999999999999991118, 9.499999999999998224 ) ) ;
#3590=ORIENTED_EDGE ( 'NONE', *, *, #5011, .T. ) ;
#3595=LINE ( 'NONE', #266, #6119 ) ;
#3600=DIRECTION ( 'NONE',  ( 0.000000000000000000, 0.000000000000000000, 1.000000000000000000 ) ) ;
#3608=DIRECTION ( 'NONE',  ( 1.000000000000000000, -0.000000000000000000, -0.000000000000000000 ) ) ;
#3620=VECTOR ( 'NONE', #4636, 1000.000000000000114 ) ;
#3622=VERTEX_POINT ( 'NONE', #6583 ) ;
#3633=EDGE_CURVE ( 'NONE', #2855, #4621, #177, .T. ) ;
#3635=CARTESIAN_POINT ( 'NONE',  ( 50.00000000000000000, 1.734723475976807094E-15, -12.50000000000000000 ) ) ;
#3637=CARTESIAN_POINT ( 'NONE',  ( 50.00000000000000000, -9.999999999999994671, 0.000000000000000000 ) ) ;
#3661=EDGE_CURVE ( 'NONE', #5740, #1450, #5994, .T. ) ;
#3670=VECTOR ( 'NONE', #3346, 1000.000000000000000 ) ;
#3673=DIRECTION ( 'NONE',  ( -0.000000000000000000, 1.000000000000000000, 2.168404344971010347E-16 ) ) ;
#3674=ORIENTED_EDGE ( 'NONE', *, *, #7070, .F. ) ;
#3691=FACE_BOUND ( 'NONE', #8047, .T. ) ;
#3705=VERTEX_POINT ( 'NONE', #4097 ) ;
#3719=DIRECTION ( 'NONE',  ( 1.000000000000000000, 0.000000000000000000, -0.000000000000000000 ) ) ;
#3756=VECTOR ( 'NONE', #6457, 1000.000000000000000 ) ;
#3757=CARTESIAN_POINT ( 'NONE',  ( 50.00000000000000000, -9.999999999999994671, -1.500000000000000666 ) ) ;
#3772=EDGE_LOOP ( 'NONE', ( #832, #2183, #6164, #6972 ) ) ;
#3812=VECTOR ( 'NONE', #2356, 1000.000000000000000 ) ;
#3814=ORIENTED_EDGE ( 'NONE', *, *, #2898, .T. ) ;
#3826=CIRCLE ( 'NONE', #5572, 1.499999999999996225 ) ;
#3828=EDGE_CURVE ( 'NONE', #6779, #2259, #5400, .T. ) ;
#3832=VERTEX_POINT ( 'NONE', #4764 ) ;
#3898=LINE ( 'NONE', #1203, #1812 ) ;
#3899=AXIS2_PLACEMENT_3D ( 'NONE', #5395, #2912, #6741 ) ;
#3905=CARTESIAN_POINT ( 'NONE',  ( 45.00000000000000000, -15.00000000000000355, 9.500000000000000000 ) ) ;
#3913=CYLINDRICAL_SURFACE ( 'NONE', #5228, 4.999999999999999112 ) ;
#3916=VERTEX_POINT ( 'NONE', #2611 ) ;
#3931=FACE_OUTER_BOUND ( 'NONE', #4353, .T. ) ;
#3935=EDGE_CURVE ( 'NONE', #7792, #348, #8215, .T. ) ;
#3936=ORIENTED_EDGE ( 'NONE', *, *, #7958, .T. ) ;
#3951=AXIS2_PLACEMENT_3D ( 'NONE', #2780, #4832, #2150 ) ;
#3963=EDGE_CURVE ( 'NONE', #6901, #2088, #6506, .T. ) ;
#3967=CYLINDRICAL_SURFACE ( 'NONE', #129, 1.500000000000000666 ) ;
#3973=DIRECTION ( 'NONE',  ( -1.000000000000000000, -0.000000000000000000, 0.000000000000000000 ) ) ;
#3976=EDGE_CURVE ( 'NONE', #2390, #4159, #3243, .T. ) ;
#3983=CARTESIAN_POINT ( 'NONE',  ( 46.49999999999999289, -14.99999999999999467, -12.50000000000000178 ) ) ;
#3988=LINE ( 'NONE', #5967, #8001 ) ;
#3998=ORIENTED_EDGE ( 'NONE', *, *, #158, .T. ) ;
#4017=EDGE_CURVE ( 'NONE', #1490, #7328, #2524, .T. ) ;
#4020=VERTEX_POINT ( 'NONE', #5672 ) ;
#4038=ORIENTED_EDGE ( 'NONE', *, *, #1289, .F. ) ;
#4039=DIRECTION ( 'NONE',  ( -0.000000000000000000, 1.000000000000000000, 2.168404344971010594E-16 ) ) ;
#4048=DIRECTION ( 'NONE',  ( 1.000000000000000000, 0.000000000000000000, 0.000000000000000000 ) ) ;
#4050=CARTESIAN_POINT ( 'NONE',  ( 40.00000000000000000, -9.999999999999992895, 4.499999999999999112 ) ) ;
#4055=CARTESIAN_POINT ( 'NONE',  ( 50.00000000000000000, -7.999999999999996447, 12.49999999999999822 ) ) ;
#4066=PLANE ( 'NONE',  #1348 ) ;
#4084=VECTOR ( 'NONE', #8201, 1000.000000000000000 ) ;
#4087=ORIENTED_EDGE ( 'NONE', *, *, #1320, .T. ) ;
#4097=CARTESIAN_POINT ( 'NONE',  ( 40.00000000000000000, -14.99999999999999112, 4.499999999999999112 ) ) ;
#4101=ORIENTED_EDGE ( 'NONE', *, *, #2898, .F. ) ;
#4104=EDGE_LOOP ( 'NONE', ( #4101, #7946, #4431, #7375, #4208 ) ) ;
#4114=ORIENTED_EDGE ( 'NONE', *, *, #328, .T. ) ;
#4137=FACE_OUTER_BOUND ( 'NONE', #1544, .T. ) ;
#4139=ORIENTED_EDGE ( 'NONE', *, *, #7958, .F. ) ;
#4159=VERTEX_POINT ( 'NONE', #6649 ) ;
#4174=PLANE ( 'NONE',  #6425 ) ;
#4179=ORIENTED_EDGE ( 'NONE', *, *, #3100, .F. ) ;
#4187=DIRECTION ( 'NONE',  ( 0.000000000000000000, 0.000000000000000000, 1.000000000000000000 ) ) ;
#4193=DIRECTION ( 'NONE',  ( 0.000000000000000000, -1.387778780781445676E-16, 1.000000000000000000 ) ) ;
#4195=DIRECTION ( 'NONE',  ( -0.000000000000000000, 1.734723475976807094E-16, -1.000000000000000000 ) ) ;
#4207=CARTESIAN_POINT ( 'NONE',  ( 50.00000000000000000, -9.999999999999991118, -10.50000000000000888 ) ) ;
#4208=ORIENTED_EDGE ( 'NONE', *, *, #5375, .T. ) ;
#4213=LINE ( 'NONE', #3586, #1451 ) ;
#4223=EDGE_CURVE ( 'NONE', #6872, #4020, #748, .T. ) ;
#4228=CIRCLE ( 'NONE', #3556, 1.500000000000000666 ) ;
#4230=LINE ( 'NONE', #3519, #2617 ) ;
#4231=VECTOR ( 'NONE', #7834, 1000.000000000000000 ) ;
#4233=SURFACE_SIDE_STYLE ('',( #1670 ) ) ;
#4235=ORIENTED_EDGE ( 'NONE', *, *, #842, .T. ) ;
#4236=DIRECTION ( 'NONE',  ( 0.000000000000000000, -1.000000000000000000, -2.775557561562891351E-16 ) ) ;
#4237=EDGE_CURVE ( 'NONE', #1673, #4574, #2190, .T. ) ;
#4238=ORIENTED_EDGE ( 'NONE', *, *, #6316, .T. ) ;
#4250=DIRECTION ( 'NONE',  ( 0.000000000000000000, 0.000000000000000000, -1.000000000000000000 ) ) ;
#4277=CARTESIAN_POINT ( 'NONE',  ( 80.00000000000000000, -7.999999999999996447, 12.49999999999999822 ) ) ;
#4286=VECTOR ( 'NONE', #3303, 1000.000000000000000 ) ;
#4290=ORIENTED_EDGE ( 'NONE', *, *, #414, .F. ) ;
#4299=( NAMED_UNIT ( * ) PLANE_ANGLE_UNIT ( ) SI_UNIT ( $, .RADIAN. ) );
#4308=DIRECTION ( 'NONE',  ( -0.000000000000000000, -8.673617379884033007E-17, -1.000000000000000000 ) ) ;
#4313=LINE ( 'NONE', #7488, #8010 ) ;
#4334=AXIS2_PLACEMENT_3D ( 'NONE', #2504, #5066, #6377 ) ;
#4339=FACE_OUTER_BOUND ( 'NONE', #7117, .T. ) ;
#4348=AXIS2_PLACEMENT_3D ( 'NONE', #5756, #3200, #7624 ) ;
#4352=AXIS2_PLACEMENT_3D ( 'NONE', #1710, #5535, #3600 ) ;
#4353=EDGE_LOOP ( 'NONE', ( #1507, #4713, #4770, #4863, #2489, #7500, #3936, #5279, #2268, #1302 ) ) ;
#4355=FACE_OUTER_BOUND ( 'NONE', #7998, .T. ) ;
#4357=ORIENTED_EDGE ( 'NONE', *, *, #3828, .F. ) ;
#4358=CARTESIAN_POINT ( 'NONE',  ( 75.00000000000000000, 1.301042606982605715E-15, -7.500000000000002665 ) ) ;
#4371=ORIENTED_EDGE ( 'NONE', *, *, #2976, .F. ) ;
#4405=EDGE_LOOP ( 'NONE', ( #4753, #1982, #4238, #5633 ) ) ;
#4408=ORIENTED_EDGE ( 'NONE', *, *, #359, .F. ) ;
#4416=CARTESIAN_POINT ( 'NONE',  ( 54.99999999999999289, 1.301042606982605715E-15, -7.500000000000002665 ) ) ;
#4429=COLOUR_RGB ( '', 0.08235294, 0.09019608, 0.10196078) ;
#4431=ORIENTED_EDGE ( 'NONE', *, *, #2789, .T. ) ;
#4432=CARTESIAN_POINT ( 'NONE',  ( 50.00000000000000000, -7.999999999999992895, -12.50000000000000178 ) ) ;
#4435=ADVANCED_FACE ( 'NONE', ( #4137 ), #852, .F. ) ;
#4437=EDGE_LOOP ( 'NONE', ( #4357, #3198, #1176, #3590 ) ) ;
#4445=CARTESIAN_POINT ( 'NONE',  ( 75.00000000000000000, 1.040834085586084848E-15, -7.500000000000003553 ) ) ;
#4451=ORIENTED_EDGE ( 'NONE', *, *, #1793, .T. ) ;
#4459=LINE ( 'NONE', #6535, #2690 ) ;
#4465=CARTESIAN_POINT ( 'NONE',  ( 50.00000000000000000, -9.999999999999994671, 1.500000000000000666 ) ) ;
#4470=CARTESIAN_POINT ( 'NONE',  ( 50.00000000000000000, -9.999999999999991118, -10.50000000000000888 ) ) ;
#4475=DIRECTION ( 'NONE',  ( -0.000000000000000000, 2.775557561562891351E-16, -1.000000000000000000 ) ) ;
#4478=ORIENTED_EDGE ( 'NONE', *, *, #328, .F. ) ;
#4493=CARTESIAN_POINT ( 'NONE',  ( 75.00000000000000000, -1.301042606982604729E-15, 7.499999999999997335 ) ) ;
#4496=EDGE_LOOP ( 'NONE', ( #4139, #2006, #2486, #6056 ) ) ;
#4504=DIRECTION ( 'NONE',  ( 1.000000000000000000, 0.000000000000000000, 0.000000000000000000 ) ) ;
#4505=DIRECTION ( 'NONE',  ( 0.000000000000000000, -2.775557561562891351E-16, 1.000000000000000000 ) ) ;
#4508=DIRECTION ( 'NONE',  ( 0.000000000000000000, 1.000000000000000000, -1.734723475976806108E-16 ) ) ;
#4511=DIRECTION ( 'NONE',  ( 1.000000000000000000, 0.000000000000000000, 0.000000000000000000 ) ) ;
#4516=ORIENTED_EDGE ( 'NONE', *, *, #3043, .F. ) ;
#4522=EDGE_CURVE ( 'NONE', #2390, #3622, #4937, .T. ) ;
#4536=ORIENTED_EDGE ( 'NONE', *, *, #2230, .F. ) ;
#4543=MANIFOLD_SOLID_BREP ( 'Cut-Extrude2', #1549 ) ;
#4548=CARTESIAN_POINT ( 'NONE',  ( 80.00000000000000000, -9.999999999999994671, 1.500000000000000666 ) ) ;
#4555=EDGE_CURVE ( 'NONE', #3832, #2974, #1701, .T. ) ;
#4557=EDGE_LOOP ( 'NONE', ( #4038, #4536, #2743, #7635 ) ) ;
#4574=VERTEX_POINT ( 'NONE', #4416 ) ;
#4575=FACE_OUTER_BOUND ( 'NONE', #1632, .T. ) ;
#4583=ADVANCED_FACE ( 'NONE', ( #424 ), #548, .T. ) ;
#4587=DIRECTION ( 'NONE',  ( 1.000000000000000000, 0.000000000000000000, 0.000000000000000000 ) ) ;
#4591=DIRECTION ( 'NONE',  ( 0.000000000000000000, -1.734723475976806108E-16, -1.000000000000000000 ) ) ;
#4603=CARTESIAN_POINT ( 'NONE',  ( 75.00000000000000000, -30.00000000000000000, 7.499999999999992006 ) ) ;
#4616=AXIS2_PLACEMENT_3D ( 'NONE', #7786, #1375, #740 ) ;
#4621=VERTEX_POINT ( 'NONE', #6200 ) ;
#4636=DIRECTION ( 'NONE',  ( 0.000000000000000000, -0.7071067811865507924, 0.7071067811865441310 ) ) ;
#4638=CARTESIAN_POINT ( 'NONE',  ( 50.00000000000000000, -19.99999999999999645, -7.500000000000006217 ) ) ;
#4647=VERTEX_POINT ( 'NONE', #3169 ) ;
#4665=ORIENTED_EDGE ( 'NONE', *, *, #4223, .F. ) ;
#4671=DIRECTION ( 'NONE',  ( 0.000000000000000000, 0.7071067811865507924, 0.7071067811865441310 ) ) ;
#4673=DIRECTION ( 'NONE',  ( 1.000000000000000000, 0.000000000000000000, 0.000000000000000000 ) ) ;
#4678=CARTESIAN_POINT ( 'NONE',  ( 50.00000000000000000, -9.999999999999994671, -1.500000000000000666 ) ) ;
#4713=ORIENTED_EDGE ( 'NONE', *, *, #6386, .T. ) ;
#4714=CARTESIAN_POINT ( 'NONE',  ( 50.00000000000000000, -20.00000000000000355, 7.499999999999996447 ) ) ;
#4720=LINE ( 'NONE', #4678, #2995 ) ;
#4736=ORIENTED_EDGE ( 'NONE', *, *, #3178, .F. ) ;
#4753=ORIENTED_EDGE ( 'NONE', *, *, #1919, .T. ) ;
#4764=CARTESIAN_POINT ( 'NONE',  ( 75.00000000000000000, -9.999999999999994671, -1.500000000000000666 ) ) ;
#4767=EDGE_CURVE ( 'NONE', #1450, #2779, #4459, .T. ) ;
#4770=ORIENTED_EDGE ( 'NONE', *, *, #3043, .T. ) ;
#4775=ORIENTED_EDGE ( 'NONE', *, *, #3828, .T. ) ;
#4784=VERTEX_POINT ( 'NONE', #3210 ) ;
#4832=DIRECTION ( 'NONE',  ( 0.000000000000000000, -0.7071067811865465735, 0.7071067811865485719 ) ) ;
#4852=DIRECTION ( 'NONE',  ( 0.000000000000000000, -1.000000000000000000, 0.000000000000000000 ) ) ;
#4858=ORIENTED_EDGE ( 'NONE', *, *, #3004, .F. ) ;
#4863=ORIENTED_EDGE ( 'NONE', *, *, #5085, .T. ) ;
#4868=DIRECTION ( 'NONE',  ( 0.000000000000000000, -0.7071067811865507924, 0.7071067811865441310 ) ) ;
#4871=( NAMED_UNIT ( * ) PLANE_ANGLE_UNIT ( ) SI_UNIT ( $, .RADIAN. ) );
#4873=ORIENTED_EDGE ( 'NONE', *, *, #3976, .F. ) ;
#4876=VERTEX_POINT ( 'NONE', #3299 ) ;
#4895=EDGE_CURVE ( 'NONE', #4784, #3705, #1393, .T. ) ;
#4898=VECTOR ( 'NONE', #7708, 1000.000000000000000 ) ;
#4900=EDGE_LOOP ( 'NONE', ( #6331, #4087, #8057, #8252 ) ) ;
#4911=CARTESIAN_POINT ( 'NONE',  ( 80.00000000000000000, -9.999999999999994671, 10.50000000000000533 ) ) ;
#4916=CARTESIAN_POINT ( 'NONE',  ( 50.00000000000000000, -1.734723475976807094E-15, 12.50000000000000000 ) ) ;
#4917=ORIENTED_EDGE ( 'NONE', *, *, #7070, .T. ) ;
#4937=LINE ( 'NONE', #3635, #2550 ) ;
#4989=( NAMED_UNIT ( * ) PLANE_ANGLE_UNIT ( ) SI_UNIT ( $, .RADIAN. ) );
#5011=EDGE_CURVE ( 'NONE', #1658, #2259, #7123, .T. ) ;
#5017=DIRECTION ( 'NONE',  ( 0.000000000000000000, -0.7071067811865507924, 0.7071067811865441310 ) ) ;
#5026=EDGE_CURVE ( 'NONE', #3622, #2855, #6147, .T. ) ;
#5047=ORIENTED_EDGE ( 'NONE', *, *, #4767, .F. ) ;
#5061=LINE ( 'NONE', #1192, #1604 ) ;
#5066=DIRECTION ( 'NONE',  ( 1.000000000000000000, 0.000000000000000000, 0.000000000000000000 ) ) ;
#5070=VERTEX_POINT ( 'NONE', #1647 ) ;
#5085=EDGE_CURVE ( 'NONE', #8159, #6872, #2161, .T. ) ;
#5088=CARTESIAN_POINT ( 'NONE',  ( 50.00000000000000000, -9.999999999999991118, 9.499999999999998224 ) ) ;
#5107=CARTESIAN_POINT ( 'NONE',  ( 45.00000000000000000, -14.99999999999999112, 9.500000000000000000 ) ) ;
#5143=CIRCLE ( 'NONE', #4334, 1.500000000000000666 ) ;
#5148=DIRECTION ( 'NONE',  ( 0.000000000000000000, 1.000000000000000000, 0.000000000000000000 ) ) ;
#5149=EDGE_CURVE ( 'NONE', #914, #5848, #7934, .T. ) ;
#5155=AXIS2_PLACEMENT_3D ( 'NONE', #876, #6565, #7924 ) ;
#5157=VECTOR ( 'NONE', #1614, 1000.000000000000000 ) ;
#5197=ORIENTED_EDGE ( 'NONE', *, *, #3240, .F. ) ;
#5211=AXIS2_PLACEMENT_3D ( 'NONE', #2001, #6460, #4511 ) ;
#5217=ORIENTED_EDGE ( 'NONE', *, *, #359, .T. ) ;
#5228=AXIS2_PLACEMENT_3D ( 'NONE', #7072, #7707, #2066 ) ;
#5242=CIRCLE ( 'NONE', #1481, 1.500000000000000666 ) ;
#5243=DIRECTION ( 'NONE',  ( 0.000000000000000000, 0.000000000000000000, -1.000000000000000000 ) ) ;
#5249=ADVANCED_FACE ( 'NONE', ( #1603 ), #5476, .T. ) ;
#5258=DIRECTION ( 'NONE',  ( -0.000000000000000000, 1.000000000000000000, 2.168404344971010347E-16 ) ) ;
#5266=EDGE_CURVE ( 'NONE', #348, #2974, #3486, .T. ) ;
#5270=CYLINDRICAL_SURFACE ( 'NONE', #7267, 5.000000000000000888 ) ;
#5279=ORIENTED_EDGE ( 'NONE', *, *, #3240, .T. ) ;
#5286=LINE ( 'NONE', #3983, #2080 ) ;
#5288=CARTESIAN_POINT ( 'NONE',  ( 50.00000000000000000, -1.734723475976807094E-15, 12.50000000000000000 ) ) ;
#5301=DIRECTION ( 'NONE',  ( 0.000000000000000000, -2.168404344971010101E-16, 1.000000000000000000 ) ) ;
#5312=FACE_OUTER_BOUND ( 'NONE', #4104, .T. ) ;
#5338=ORIENTED_EDGE ( 'NONE', *, *, #1320, .F. ) ;
#5339=CARTESIAN_POINT ( 'NONE',  ( 45.00000000000000000, -14.99999999999999467, -12.50000000000000178 ) ) ;
#5351=CIRCLE ( 'NONE', #7645, 4.999999999999999112 ) ;
#5365=EDGE_LOOP ( 'NONE', ( #5197, #6528, #5670, #8237 ) ) ;
#5371=DIRECTION ( 'NONE',  ( 0.000000000000000000, -1.000000000000000000, 0.000000000000000000 ) ) ;
#5375=EDGE_CURVE ( 'NONE', #1819, #3497, #1732, .T. ) ;
#5380=CIRCLE ( 'NONE', #7672, 1.499999999999996225 ) ;
#5394=CARTESIAN_POINT ( 'NONE',  ( 80.00000000000000000, -12.00000000000000711, 12.49999999999999822 ) ) ;
#5395=CARTESIAN_POINT ( 'NONE',  ( 75.00000000000000000, -30.00000000000000000, -7.500000000000007105 ) ) ;
#5400=LINE ( 'NONE', #7981, #5157 ) ;
#5407=DIRECTION ( 'NONE',  ( 1.000000000000000000, 0.000000000000000000, 0.000000000000000000 ) ) ;
#5436=CARTESIAN_POINT ( 'NONE',  ( 45.00000000000000000, -14.99999999999999467, 9.499999999999996447 ) ) ;
#5443=DIRECTION ( 'NONE',  ( 0.000000000000000000, 1.000000000000000000, 2.168404344971010347E-16 ) ) ;
#5450=CARTESIAN_POINT ( 'NONE',  ( 50.00000000000000000, -12.00000000000000355, -12.50000000000000178 ) ) ;
#5465=CARTESIAN_POINT ( 'NONE',  ( 80.00000000000000000, -12.00000000000000355, -12.50000000000000178 ) ) ;
#5476=PLANE ( 'NONE',  #7938 ) ;
#5482=CARTESIAN_POINT ( 'NONE',  ( 80.00000000000000000, -1.734723475976807094E-15, 12.50000000000000000 ) ) ;
#5485=VECTOR ( 'NONE', #2564, 1000.000000000000000 ) ;
#5495=FACE_BOUND ( 'NONE', #7580, .T. ) ;
#5497=DIRECTION ( 'NONE',  ( 0.000000000000000000, 0.000000000000000000, 1.000000000000000000 ) ) ;
#5499=VERTEX_POINT ( 'NONE', #3116 ) ;
#5503=VERTEX_POINT ( 'NONE', #373 ) ;
#5504=COLOUR_RGB ( '', 0.08235294, 0.09019608, 0.10196078) ;
#5517=ORIENTED_EDGE ( 'NONE', *, *, #5375, .F. ) ;
#5535=DIRECTION ( 'NONE',  ( -1.000000000000000000, -0.000000000000000000, 0.000000000000000000 ) ) ;
#5541=UNCERTAINTY_MEASURE_WITH_UNIT (LENGTH_MEASURE( 1.000000000000000082E-05 ), #1740, 'distance_accuracy_value', 'NONE');
#5543=ORIENTED_EDGE ( 'NONE', *, *, #3004, .T. ) ;
#5555=VERTEX_POINT ( 'NONE', #4493 ) ;
#5572=AXIS2_PLACEMENT_3D ( 'NONE', #5783, #7650, #11 ) ;
#5577=ADVANCED_FACE ( 'NONE', ( #618 ), #3913, .T. ) ;
#5580=DIRECTION ( 'NONE',  ( -0.000000000000000000, 1.000000000000000000, 1.387778780781445676E-16 ) ) ;
#5594=ORIENTED_EDGE ( 'NONE', *, *, #414, .T. ) ;
#5600=CARTESIAN_POINT ( 'NONE',  ( 50.00000000000000000, -20.00000000000000355, 9.499999999999998224 ) ) ;
#5603=CARTESIAN_POINT ( 'NONE',  ( 50.00000000000000000, -7.999999999999992895, -12.50000000000000178 ) ) ;
#5605=PLANE ( 'NONE',  #7729 ) ;
#5614=CARTESIAN_POINT ( 'NONE',  ( 80.00000000000000000, 1.734723475976807094E-15, -12.50000000000000000 ) ) ;
#5633=ORIENTED_EDGE ( 'NONE', *, *, #5827, .F. ) ;
#5660=CARTESIAN_POINT ( 'NONE',  ( 50.00000000000000000, -19.99999999999999645, -12.50000000000000355 ) ) ;
#5670=ORIENTED_EDGE ( 'NONE', *, *, #903, .T. ) ;
#5672=CARTESIAN_POINT ( 'NONE',  ( 80.00000000000000000, -19.99999999999999645, -12.50000000000000355 ) ) ;
#5676=EDGE_CURVE ( 'NONE', #4159, #2855, #3199, .T. ) ;
#5695=CIRCLE ( 'NONE', #2762, 1.499999999999994449 ) ;
#5704=CARTESIAN_POINT ( 'NONE',  ( 50.00000000000000000, -20.00000000000000355, 12.49999999999999645 ) ) ;
#5713=ORIENTED_EDGE ( 'NONE', *, *, #6870, .F. ) ;
#5728=DIRECTION ( 'NONE',  ( 1.000000000000000000, 0.000000000000000000, 0.000000000000000000 ) ) ;
#5732=DIRECTION ( 'NONE',  ( -0.000000000000000000, 0.7071067811865484609, -0.7071067811865465735 ) ) ;
#5739=PRODUCT_CONTEXT ( 'NONE', #992, 'mechanical' ) ;
#5740=VERTEX_POINT ( 'NONE', #7794 ) ;
#5756=CARTESIAN_POINT ( 'NONE',  ( 54.99999999999999289, -9.999999999999994671, 0.000000000000000000 ) ) ;
#5772=DIRECTION ( 'NONE',  ( 0.000000000000000000, -1.000000000000000000, -2.168404344971010347E-16 ) ) ;
#5781=VERTEX_POINT ( 'NONE', #2026 ) ;
#5783=CARTESIAN_POINT ( 'NONE',  ( 45.00000000000000000, -14.99999999999999467, 4.499999999999999112 ) ) ;
#5785=ADVANCED_FACE ( 'NONE', ( #4575, #7159 ), #6400, .T. ) ;
#5801=ORIENTED_EDGE ( 'NONE', *, *, #1229, .F. ) ;
#5813=VECTOR ( 'NONE', #7178, 1000.000000000000000 ) ;
#5814=CARTESIAN_POINT ( 'NONE',  ( 50.00000000000000000, -9.999999999999994671, 10.50000000000000533 ) ) ;
#5827=EDGE_CURVE ( 'NONE', #5503, #1673, #7839, .T. ) ;
#5829=CIRCLE ( 'NONE', #700, 4.999999999999999112 ) ;
#5834=DIRECTION ( 'NONE',  ( -0.000000000000000000, 0.7071067811865507924, 0.7071067811865441310 ) ) ;
#5848=VERTEX_POINT ( 'NONE', #2523 ) ;
#5874=CARTESIAN_POINT ( 'NONE',  ( 80.00000000000000000, -9.999999999999991118, -10.50000000000000888 ) ) ;
#5877=CARTESIAN_POINT ( 'NONE',  ( 75.00000000000000000, -9.999999999999994671, 0.000000000000000000 ) ) ;
#5889=VERTEX_POINT ( 'NONE', #1508 ) ;
#5904=CARTESIAN_POINT ( 'NONE',  ( 50.00000000000000000, -7.999999999999992895, -12.50000000000000178 ) ) ;
#5920=DIRECTION ( 'NONE',  ( 1.000000000000000000, 0.000000000000000000, 0.000000000000000000 ) ) ;
#5933=CARTESIAN_POINT ( 'NONE',  ( 80.00000000000000000, -19.99999999999999645, -12.50000000000000355 ) ) ;
#5942=EDGE_CURVE ( 'NONE', #4020, #5889, #791, .T. ) ;
#5944=DIRECTION ( 'NONE',  ( 0.000000000000000000, -3.469446951953615175E-16, -1.000000000000000000 ) ) ;
#5963=ADVANCED_FACE ( 'NONE', ( #7964 ), #957, .T. ) ;
#5967=CARTESIAN_POINT ( 'NONE',  ( 50.00000000000000000, -7.999999999999996447, 12.49999999999999822 ) ) ;
#5987=ORIENTED_EDGE ( 'NONE', *, *, #4522, .T. ) ;
#5988=DIRECTION ( 'NONE',  ( 0.000000000000000000, -1.000000000000000000, -2.168404344971009854E-16 ) ) ;
#5994=LINE ( 'NONE', #4055, #5813 ) ;
#6000=ADVANCED_FACE ( 'NONE', ( #3413 ), #7282, .F. ) ;
#6009=ORIENTED_EDGE ( 'NONE', *, *, #7387, .T. ) ;
#6031=ADVANCED_FACE ( 'NONE', ( #6648 ), #7361, .T. ) ;
#6038=ORIENTED_EDGE ( 'NONE', *, *, #3633, .F. ) ;
#6044=FACE_OUTER_BOUND ( 'NONE', #6928, .T. ) ;
#6045=AXIS2_PLACEMENT_3D ( 'NONE', #678, #4591, #4508 ) ;
#6049=CARTESIAN_POINT ( 'NONE',  ( 40.00000000000000000, -9.999999999999992895, 4.499999999999999112 ) ) ;
#6053=DIRECTION ( 'NONE',  ( -0.000000000000000000, 2.775557561562891351E-16, -1.000000000000000000 ) ) ;
#6056=ORIENTED_EDGE ( 'NONE', *, *, #3253, .T. ) ;
#6057=FACE_OUTER_BOUND ( 'NONE', #7776, .T. ) ;
#6071=CARTESIAN_POINT ( 'NONE',  ( 50.00000000000000000, -9.999999999999994671, 0.000000000000000000 ) ) ;
#6080=CARTESIAN_POINT ( 'NONE',  ( 50.00000000000000000, -9.999999999999992895, 4.499999999999999112 ) ) ;
#6083=ORIENTED_EDGE ( 'NONE', *, *, #1752, .F. ) ;
#6092=ADVANCED_FACE ( 'NONE', ( #6057 ), #6094, .T. ) ;
#6093=ORIENTED_EDGE ( 'NONE', *, *, #1520, .F. ) ;
#6094=PLANE ( 'NONE',  #3951 ) ;
#6113=PLANE ( 'NONE',  #637 ) ;
#6116=VECTOR ( 'NONE', #6053, 1000.000000000000000 ) ;
#6118=VERTEX_POINT ( 'NONE', #2232 ) ;
#6119=VECTOR ( 'NONE', #5407, 1000.000000000000000 ) ;
#6127=CARTESIAN_POINT ( 'NONE',  ( 50.00000000000000000, -12.00000000000000711, 12.49999999999999822 ) ) ;
#6133=CARTESIAN_POINT ( 'NONE',  ( 54.99999999999999289, -1.301042606982604729E-15, 7.499999999999997335 ) ) ;
#6147=LINE ( 'NONE', #6659, #6174 ) ;
#6164=ORIENTED_EDGE ( 'NONE', *, *, #7782, .T. ) ;
#6170=PRESENTATION_STYLE_ASSIGNMENT (( #518 ) ) ;
#6174=VECTOR ( 'NONE', #6617, 1000.000000000000000 ) ;
#6177=ORIENTED_EDGE ( 'NONE', *, *, #226, .F. ) ;
#6199=EDGE_CURVE ( 'NONE', #5781, #1490, #6807, .T. ) ;
#6200=CARTESIAN_POINT ( 'NONE',  ( 80.00000000000000000, -1.734723475976807094E-15, 12.50000000000000000 ) ) ;
#6210=CARTESIAN_POINT ( 'NONE',  ( 45.00000000000000000, -14.99999999999999289, 4.499999999999999112 ) ) ;
#6219=ORIENTED_EDGE ( 'NONE', *, *, #7387, .F. ) ;
#6231=VERTEX_POINT ( 'NONE', #5660 ) ;
#6236=VECTOR ( 'NONE', #4195, 1000.000000000000000 ) ;
#6262=PLANE ( 'NONE',  #2091 ) ;
#6275=ORIENTED_EDGE ( 'NONE', *, *, #611, .T. ) ;
#6287=ORIENTED_EDGE ( 'NONE', *, *, #6316, .F. ) ;
#6316=EDGE_CURVE ( 'NONE', #5555, #1673, #1081, .T. ) ;
#6320=DIRECTION ( 'NONE',  ( 1.000000000000000000, 0.000000000000000000, 0.000000000000000000 ) ) ;
#6329=VECTOR ( 'NONE', #781, 1000.000000000000000 ) ;
#6331=ORIENTED_EDGE ( 'NONE', *, *, #2092, .F. ) ;
#6332=EDGE_CURVE ( 'NONE', #6231, #4020, #2978, .T. ) ;
#6377=DIRECTION ( 'NONE',  ( 0.000000000000000000, 0.000000000000000000, -1.000000000000000000 ) ) ;
#6378=VECTOR ( 'NONE', #703, 1000.000000000000000 ) ;
#6386=EDGE_CURVE ( 'NONE', #6524, #2779, #2473, .T. ) ;
#6387=VERTEX_POINT ( 'NONE', #443 ) ;
#6400=PLANE ( 'NONE',  #8328 ) ;
#6413=CARTESIAN_POINT ( 'NONE',  ( 50.00000000000000000, -1.734723475976807094E-15, 12.50000000000000000 ) ) ;
#6422=EDGE_LOOP ( 'NONE', ( #2365, #4371 ) ) ;
#6425=AXIS2_PLACEMENT_3D ( 'NONE', #299, #2876, #5443 ) ;
#6437=ORIENTED_EDGE ( 'NONE', *, *, #5149, .F. ) ;
#6447=VECTOR ( 'NONE', #2, 1000.000000000000000 ) ;
#6448=VECTOR ( 'NONE', #7203, 1000.000000000000000 ) ;
#6457=DIRECTION ( 'NONE',  ( -0.000000000000000000, 1.000000000000000000, 1.734723475976807094E-16 ) ) ;
#6460=DIRECTION ( 'NONE',  ( -0.000000000000000000, -0.000000000000000000, 1.000000000000000000 ) ) ;
#6461=DIRECTION ( 'NONE',  ( 0.000000000000000000, 0.000000000000000000, -1.000000000000000000 ) ) ;
#6499=DIRECTION ( 'NONE',  ( 0.000000000000000000, 0.000000000000000000, 1.000000000000000000 ) ) ;
#6502=SHAPE_REPRESENTATION ( 'jaw base', ( #2840 ), #7820 ) ;
#6506=CIRCLE ( 'NONE', #4348, 1.500000000000000666 ) ;
#6524=VERTEX_POINT ( 'NONE', #7654 ) ;
#6528=ORIENTED_EDGE ( 'NONE', *, *, #3253, .F. ) ;
#6535=CARTESIAN_POINT ( 'NONE',  ( 50.00000000000000000, -9.999999999999994671, 10.50000000000000533 ) ) ;
#6548=ORIENTED_EDGE ( 'NONE', *, *, #694, .F. ) ;
#6565=DIRECTION ( 'NONE',  ( 0.000000000000000000, 2.168404344971010594E-16, -1.000000000000000000 ) ) ;
#6579=AXIS2_PLACEMENT_3D ( 'NONE', #5436, #3580, #4048 ) ;
#6583=CARTESIAN_POINT ( 'NONE',  ( 50.00000000000000000, 1.734723475976807094E-15, -12.50000000000000000 ) ) ;
#6605=ORIENTED_EDGE ( 'NONE', *, *, #2976, .T. ) ;
#6617=DIRECTION ( 'NONE',  ( 1.000000000000000000, 0.000000000000000000, 0.000000000000000000 ) ) ;
#6622=FACE_OUTER_BOUND ( 'NONE', #1040, .T. ) ;
#6625=EDGE_LOOP ( 'NONE', ( #6038, #7688, #1116, #482 ) ) ;
#6645=CIRCLE ( 'NONE', #1538, 1.500000000000000666 ) ;
#6648=FACE_OUTER_BOUND ( 'NONE', #2999, .T. ) ;
#6649=CARTESIAN_POINT ( 'NONE',  ( 80.00000000000000000, -7.999999999999992895, -12.50000000000000178 ) ) ;
#6659=CARTESIAN_POINT ( 'NONE',  ( 50.00000000000000000, 1.734723475976807094E-15, -12.50000000000000000 ) ) ;
#6665=DIRECTION ( 'NONE',  ( 1.000000000000000000, -0.000000000000000000, -0.000000000000000000 ) ) ;
#6667=DIRECTION ( 'NONE',  ( 1.000000000000000000, 0.000000000000000000, 0.000000000000000000 ) ) ;
#6677=CARTESIAN_POINT ( 'NONE',  ( 80.00000000000000000, -12.00000000000000711, 12.49999999999999822 ) ) ;
#6680=ORIENTED_EDGE ( 'NONE', *, *, #8250, .F. ) ;
#6713=EDGE_LOOP ( 'NONE', ( #8200, #4235, #3438, #6730 ) ) ;
#6723=ORIENTED_EDGE ( 'NONE', *, *, #5676, .F. ) ;
#6730=ORIENTED_EDGE ( 'NONE', *, *, #3356, .T. ) ;
#6738=ORIENTED_EDGE ( 'NONE', *, *, #694, .T. ) ;
#6740=ORIENTED_EDGE ( 'NONE', *, *, #2370, .F. ) ;
#6741=DIRECTION ( 'NONE',  ( 0.000000000000000000, 0.000000000000000000, -1.000000000000000000 ) ) ;
#6758=CARTESIAN_POINT ( 'NONE',  ( 80.00000000000000000, -9.999999999999994671, -1.500000000000000666 ) ) ;
#6762=ORIENTED_EDGE ( 'NONE', *, *, #8112, .F. ) ;
#6763=DIRECTION ( 'NONE',  ( 0.000000000000000000, -2.775557561562891351E-16, 1.000000000000000000 ) ) ;
#6768=ORIENTED_EDGE ( 'NONE', *, *, #43, .T. ) ;
#6774=EDGE_CURVE ( 'NONE', #4647, #1658, #5286, .T. ) ;
#6779=VERTEX_POINT ( 'NONE', #1574 ) ;
#6783=DIRECTION ( 'NONE',  ( 1.000000000000000000, 0.000000000000000000, 0.000000000000000000 ) ) ;
#6786=DIRECTION ( 'NONE',  ( -0.000000000000000000, 3.469446951953615175E-16, 1.000000000000000000 ) ) ;
#6789=VECTOR ( 'NONE', #3608, 1000.000000000000000 ) ;
#6805=CARTESIAN_POINT ( 'NONE',  ( 54.99999999999999289, -9.999999999999994671, 1.500000000000000666 ) ) ;
#6807=LINE ( 'NONE', #7490, #8260 ) ;
#6810=EDGE_CURVE ( 'NONE', #7328, #1819, #7826, .T. ) ;
#6827=VECTOR ( 'NONE', #1612, 1000.000000000000000 ) ;
#6843=VERTEX_POINT ( 'NONE', #344 ) ;
#6845=AXIS2_PLACEMENT_3D ( 'NONE', #8137, #1857, #4250 ) ;
#6846=CARTESIAN_POINT ( 'NONE',  ( 50.00000000000000000, -9.999999999999991118, -10.50000000000000888 ) ) ;
#6850=CARTESIAN_POINT ( 'NONE',  ( 50.00000000000000000, -19.99999999999999645, -12.50000000000000355 ) ) ;
#6857=VECTOR ( 'NONE', #5834, 1000.000000000000114 ) ;
#6870=EDGE_CURVE ( 'NONE', #6231, #4876, #7431, .T. ) ;
#6871=PRESENTATION_STYLE_ASSIGNMENT (( #2998 ) ) ;
#6872=VERTEX_POINT ( 'NONE', #3512 ) ;
#6901=VERTEX_POINT ( 'NONE', #305 ) ;
#6905=AXIS2_PLACEMENT_3D ( 'NONE', #3434, #6667, #1022 ) ;
#6913=SURFACE_SIDE_STYLE ('',( #6999 ) ) ;
#6915=VERTEX_POINT ( 'NONE', #1660 ) ;
#6922=AXIS2_PLACEMENT_3D ( 'NONE', #4916, #5580, #4193 ) ;
#6928=EDGE_LOOP ( 'NONE', ( #5801, #6740, #4114, #6275 ) ) ;
#6955=ORIENTED_EDGE ( 'NONE', *, *, #4895, .F. ) ;
#6972=ORIENTED_EDGE ( 'NONE', *, *, #1793, .F. ) ;
#6999=SURFACE_STYLE_FILL_AREA ( #8184 ) ;
#7015=ADVANCED_FACE ( 'NONE', ( #3357 ), #1063, .F. ) ;
#7017=ORIENTED_EDGE ( 'NONE', *, *, #5942, .F. ) ;
#7035=EDGE_CURVE ( 'NONE', #914, #5555, #2055, .T. ) ;
#7041=CARTESIAN_POINT ( 'NONE',  ( 50.00000000000000000, -9.999999999999994671, 10.50000000000000533 ) ) ;
#7070=EDGE_CURVE ( 'NONE', #2088, #6901, #6645, .T. ) ;
#7072=CARTESIAN_POINT ( 'NONE',  ( 45.00000000000000000, -14.99999999999999467, 5.204170427930420494E-15 ) ) ;
#7075=ORIENTED_EDGE ( 'NONE', *, *, #1919, .F. ) ;
#7096=ORIENTED_EDGE ( 'NONE', *, *, #734, .T. ) ;
#7115=DIRECTION ( 'NONE',  ( 1.000000000000000000, 0.000000000000000000, 0.000000000000000000 ) ) ;
#7117=EDGE_LOOP ( 'NONE', ( #4516, #5047, #5217, #789 ) ) ;
#7123=CIRCLE ( 'NONE', #6579, 1.499999999999994449 ) ;
#7128=FACE_OUTER_BOUND ( 'NONE', #4557, .T. ) ;
#7130=ADVANCED_FACE ( 'NONE', ( #4339 ), #5605, .T. ) ;
#7132=CYLINDRICAL_SURFACE ( 'NONE', #7617, 1.500000000000000666 ) ;
#7140=STYLED_ITEM ( 'NONE', ( #6170 ), #3095 ) ;
#7159=FACE_BOUND ( 'NONE', #2302, .T. ) ;
#7178=DIRECTION ( 'NONE',  ( 0.000000000000000000, -0.7071067811865484609, -0.7071067811865465735 ) ) ;
#7203=DIRECTION ( 'NONE',  ( -0.000000000000000000, 1.000000000000000000, 1.734723475976807094E-16 ) ) ;
#7220=DIRECTION ( 'NONE',  ( 1.000000000000000000, 0.000000000000000000, 0.000000000000000000 ) ) ;
#7225=ORIENTED_EDGE ( 'NONE', *, *, #6386, .F. ) ;
#7261=STYLED_ITEM ( 'NONE', ( #6871 ), #4543 ) ;
#7262=ORIENTED_EDGE ( 'NONE', *, *, #3100, .T. ) ;
#7267=AXIS2_PLACEMENT_3D ( 'NONE', #758, #4505, #3255 ) ;
#7270=ADVANCED_FACE ( 'NONE', ( #2039 ), #3967, .F. ) ;
#7273=FACE_OUTER_BOUND ( 'NONE', #4900, .T. ) ;
#7282=CYLINDRICAL_SURFACE ( 'NONE', #1804, 1.499999999999994449 ) ;
#7294=ADVANCED_FACE ( 'NONE', ( #7128 ), #5270, .T. ) ;
#7302=UNCERTAINTY_MEASURE_WITH_UNIT (LENGTH_MEASURE( 1.000000000000000082E-05 ), #2972, 'distance_accuracy_value', 'NONE');
#7316=ORIENTED_EDGE ( 'NONE', *, *, #4237, .F. ) ;
#7320=VECTOR ( 'NONE', #2342, 1000.000000000000000 ) ;
#7324=ORIENTED_EDGE ( 'NONE', *, *, #5026, .T. ) ;
#7325=DIRECTION ( 'NONE',  ( 1.000000000000000000, 0.000000000000000000, 0.000000000000000000 ) ) ;
#7328=VERTEX_POINT ( 'NONE', #2578 ) ;
#7342=FACE_OUTER_BOUND ( 'NONE', #968, .T. ) ;
#7347=DIRECTION ( 'NONE',  ( -0.000000000000000000, 1.000000000000000000, 2.168404344971010594E-16 ) ) ;
#7359=ORIENTED_EDGE ( 'NONE', *, *, #4017, .F. ) ;
#7360=ORIENTED_EDGE ( 'NONE', *, *, #3963, .T. ) ;
#7361=PLANE ( 'NONE',  #5155 ) ;
#7375=ORIENTED_EDGE ( 'NONE', *, *, #2092, .T. ) ;
#7387=EDGE_CURVE ( 'NONE', #7949, #6872, #3340, .T. ) ;
#7398=CARTESIAN_POINT ( 'NONE',  ( 45.00000000000000000, -14.99999999999999467, 9.499999999999996447 ) ) ;
#7407=LINE ( 'NONE', #1715, #2624 ) ;
#7424=PLANE ( 'NONE',  #3899 ) ;
#7427=DIRECTION ( 'NONE',  ( 0.000000000000000000, 1.734723475976807094E-16, -1.000000000000000000 ) ) ;
#7431=LINE ( 'NONE', #5450, #7869 ) ;
#7435=CARTESIAN_POINT ( 'NONE',  ( 45.00000000000000000, -9.999999999999992895, 4.499999999999999112 ) ) ;
#7443=FILL_AREA_STYLE_COLOUR ( '', #4429 ) ;
#7472=DIRECTION ( 'NONE',  ( 0.000000000000000000, -0.7071067811865465735, -0.7071067811865485719 ) ) ;
#7488=CARTESIAN_POINT ( 'NONE',  ( 50.00000000000000000, -12.00000000000000711, 12.49999999999999822 ) ) ;
#7490=CARTESIAN_POINT ( 'NONE',  ( 40.00000000000000000, -19.99999999999999645, 9.500000000000000000 ) ) ;
#7500=ORIENTED_EDGE ( 'NONE', *, *, #5942, .T. ) ;
#7511=FILL_AREA_STYLE_COLOUR ( '', #5504 ) ;
#7519=CARTESIAN_POINT ( 'NONE',  ( 50.00000000000000000, -9.999999999999994671, 0.000000000000000000 ) ) ;
#7524=ADVANCED_FACE ( 'NONE', ( #2751, #5312 ), #7895, .F. ) ;
#7551=ORIENTED_EDGE ( 'NONE', *, *, #1060, .F. ) ;
#7552=DIRECTION ( 'NONE',  ( 0.000000000000000000, 0.000000000000000000, 1.000000000000000000 ) ) ;
#7580=EDGE_LOOP ( 'NONE', ( #2107, #3674 ) ) ;
#7591=DIRECTION ( 'NONE',  ( 0.000000000000000000, 0.7071067811865485719, -0.7071067811865465735 ) ) ;
#7592=ORIENTED_EDGE ( 'NONE', *, *, #3535, .F. ) ;
#7617=AXIS2_PLACEMENT_3D ( 'NONE', #2671, #5728, #2539 ) ;
#7621=ADVANCED_FACE ( 'NONE', ( #845, #889 ), #7424, .F. ) ;
#7624=DIRECTION ( 'NONE',  ( 0.000000000000000000, 0.000000000000000000, 1.000000000000000000 ) ) ;
#7635=ORIENTED_EDGE ( 'NONE', *, *, #4895, .T. ) ;
#7645=AXIS2_PLACEMENT_3D ( 'NONE', #3543, #1526, #4852 ) ;
#7650=DIRECTION ( 'NONE',  ( 0.000000000000000000, 8.673617379884033007E-17, 1.000000000000000000 ) ) ;
#7654=CARTESIAN_POINT ( 'NONE',  ( 80.00000000000000000, -7.999999999999996447, 12.49999999999999822 ) ) ;
#7672=AXIS2_PLACEMENT_3D ( 'NONE', #314, #3361, #5371 ) ;
#7688=ORIENTED_EDGE ( 'NONE', *, *, #5026, .F. ) ;
#7706=ORIENTED_EDGE ( 'NONE', *, *, #903, .F. ) ;
#7707=DIRECTION ( 'NONE',  ( 0.000000000000000000, 3.469446951953615175E-16, 1.000000000000000000 ) ) ;
#7708=DIRECTION ( 'NONE',  ( -0.000000000000000000, 1.000000000000000000, -1.734723475976806108E-16 ) ) ;
#7710=ORIENTED_EDGE ( 'NONE', *, *, #3440, .T. ) ;
#7726=CYLINDRICAL_SURFACE ( 'NONE', #5211, 1.499999999999994449 ) ;
#7729=AXIS2_PLACEMENT_3D ( 'NONE', #7041, #1910, #5017 ) ;
#7733=VECTOR ( 'NONE', #523, 1000.000000000000000 ) ;
#7752=CARTESIAN_POINT ( 'NONE',  ( 50.00000000000000000, -9.999999999999994671, 1.500000000000000666 ) ) ;
#7775=( NAMED_UNIT ( * ) SI_UNIT ( $, .STERADIAN. ) SOLID_ANGLE_UNIT ( ) );
#7776=EDGE_LOOP ( 'NONE', ( #7225, #561, #3454, #1207 ) ) ;
#7782=EDGE_CURVE ( 'NONE', #4574, #1966, #2285, .T. ) ;
#7786=CARTESIAN_POINT ( 'NONE',  ( 75.00000000000000000, -9.999999999999994671, 0.000000000000000000 ) ) ;
#7792=VERTEX_POINT ( 'NONE', #3501 ) ;
#7794=CARTESIAN_POINT ( 'NONE',  ( 50.00000000000000000, -7.999999999999996447, 12.49999999999999822 ) ) ;
#7797=EDGE_LOOP ( 'NONE', ( #6287, #3224, #3331, #7316 ) ) ;
#7805=EDGE_CURVE ( 'NONE', #6387, #6915, #5242, .T. ) ;
#7820=( GEOMETRIC_REPRESENTATION_CONTEXT ( 3 ) GLOBAL_UNCERTAINTY_ASSIGNED_CONTEXT ( ( #3433 ) ) GLOBAL_UNIT_ASSIGNED_CONTEXT ( ( #1797, #4871, #1712 ) ) REPRESENTATION_CONTEXT ( 'NONE', 'WORKASPACE' ) );
#7822=ORIENTED_EDGE ( 'NONE', *, *, #3661, .F. ) ;
#7826=LINE ( 'NONE', #6080, #1122 ) ;
#7834=DIRECTION ( 'NONE',  ( -0.000000000000000000, 1.000000000000000000, 1.734723475976807094E-16 ) ) ;
#7838=EDGE_LOOP ( 'NONE', ( #3083, #8032 ) ) ;
#7839=LINE ( 'NONE', #1258, #6448 ) ;
#7854=FACE_BOUND ( 'NONE', #6422, .T. ) ;
#7869=VECTOR ( 'NONE', #7347, 1000.000000000000000 ) ;
#7878=CARTESIAN_POINT ( 'NONE',  ( 54.99999999999999289, -30.00000000000000000, 7.499999999999992006 ) ) ;
#7884=DIRECTION ( 'NONE',  ( -0.000000000000000000, -0.000000000000000000, 1.000000000000000000 ) ) ;
#7895=PLANE ( 'NONE',  #397 ) ;
#7913=DIRECTION ( 'NONE',  ( 0.000000000000000000, -1.000000000000000000, -1.734723475976807094E-16 ) ) ;
#7922=AXIS2_PLACEMENT_3D ( 'NONE', #5877, #1419, #2733 ) ;
#7924=DIRECTION ( 'NONE',  ( 0.000000000000000000, 1.000000000000000000, 2.168404344971010594E-16 ) ) ;
#7933=EDGE_LOOP ( 'NONE', ( #6762, #4775, #6605, #1244 ) ) ;
#7934=LINE ( 'NONE', #4714, #2947 ) ;
#7938=AXIS2_PLACEMENT_3D ( 'NONE', #4207, #1013, #4671 ) ;
#7946=ORIENTED_EDGE ( 'NONE', *, *, #1289, .T. ) ;
#7949=VERTEX_POINT ( 'NONE', #5704 ) ;
#7950=VECTOR ( 'NONE', #4673, 1000.000000000000000 ) ;
#7958=EDGE_CURVE ( 'NONE', #5889, #6843, #2688, .T. ) ;
#7964=FACE_OUTER_BOUND ( 'NONE', #76, .T. ) ;
#7981=CARTESIAN_POINT ( 'NONE',  ( 43.50000000000000711, -14.99999999999999467, -12.50000000000000178 ) ) ;
#7996=VECTOR ( 'NONE', #7115, 1000.000000000000000 ) ;
#7998=EDGE_LOOP ( 'NONE', ( #1827, #858, #3814, #641, #519, #4665, #6219, #5594 ) ) ;
#8001=VECTOR ( 'NONE', #784, 1000.000000000000000 ) ;
#8010=VECTOR ( 'NONE', #8161, 1000.000000000000000 ) ;
#8032=ORIENTED_EDGE ( 'NONE', *, *, #8112, .T. ) ;
#8047=EDGE_LOOP ( 'NONE', ( #7075, #7551, #6093, #6437 ) ) ;
#8053=AXIS2_PLACEMENT_3D ( 'NONE', #2675, #3973, #6499 ) ;
#8056=DIRECTION ( 'NONE',  ( -1.000000000000000000, 0.000000000000000000, 0.000000000000000000 ) ) ;
#8057=ORIENTED_EDGE ( 'NONE', *, *, #3535, .T. ) ;
#8065=PRODUCT_DEFINITION_CONTEXT ( 'detailed design', #1421, 'design' ) ;
#8067=EDGE_LOOP ( 'NONE', ( #6548, #1003 ) ) ;
#8070=VECTOR ( 'NONE', #5988, 1000.000000000000000 ) ;
#8076=DIRECTION ( 'NONE',  ( 1.387778780781445478E-15, -1.000000000000000000, 0.000000000000000000 ) ) ;
#8084=EDGE_CURVE ( 'NONE', #3622, #3916, #148, .T. ) ;
#8112=EDGE_CURVE ( 'NONE', #6779, #4647, #5380, .T. ) ;
#8120=CARTESIAN_POINT ( 'NONE',  ( 0.000000000000000000, 0.000000000000000000, 0.000000000000000000 ) ) ;
#8137=CARTESIAN_POINT ( 'NONE',  ( 80.00000000000000000, -9.999999999999994671, 0.000000000000000000 ) ) ;
#8159=VERTEX_POINT ( 'NONE', #6677 ) ;
#8161=DIRECTION ( 'NONE',  ( 1.000000000000000000, 0.000000000000000000, 0.000000000000000000 ) ) ;
#8184=FILL_AREA_STYLE ('',( #7511 ) ) ;
#8193=CARTESIAN_POINT ( 'NONE',  ( 80.00000000000000000, -9.999999999999994671, 10.50000000000000533 ) ) ;
#8198=LINE ( 'NONE', #2430, #6789 ) ;
#8199=PRODUCT_DEFINITION_FORMATION_WITH_SPECIFIED_SOURCE ( 'ANY', '', #1716, .NOT_KNOWN. ) ;
#8200=ORIENTED_EDGE ( 'NONE', *, *, #3935, .F. ) ;
#8201=DIRECTION ( 'NONE',  ( 0.000000000000000000, -0.7071067811865484609, -0.7071067811865465735 ) ) ;
#8204=ADVANCED_FACE ( 'NONE', ( #192 ), #2771, .F. ) ;
#8210=AXIS2_PLACEMENT_3D ( 'NONE', #2894, #2852, #7913 ) ;
#8213=ORIENTED_EDGE ( 'NONE', *, *, #3178, .T. ) ;
#8215=LINE ( 'NONE', #7752, #3143 ) ;
#8224=DIRECTION ( 'NONE',  ( 1.000000000000000000, 0.000000000000000000, 0.000000000000000000 ) ) ;
#8233=DIRECTION ( 'NONE',  ( 1.000000000000000000, 0.000000000000000000, 0.000000000000000000 ) ) ;
#8237=ORIENTED_EDGE ( 'NONE', *, *, #3976, .T. ) ;
#8250=EDGE_CURVE ( 'NONE', #4876, #1902, #1499, .T. ) ;
#8252=ORIENTED_EDGE ( 'NONE', *, *, #6810, .T. ) ;
#8253=CARTESIAN_POINT ( 'NONE',  ( 50.00000000000000000, -9.999999999999992895, 4.499999999999999112 ) ) ;
#8260=VECTOR ( 'NONE', #1166, 1000.000000000000000 ) ;
#8309=PRODUCT_DEFINITION_SHAPE ( 'NONE', 'NONE',  #1135 ) ;
#8313=ADVANCED_FACE ( 'NONE', ( #7273 ), #4066, .F. ) ;
#8328=AXIS2_PLACEMENT_3D ( 'NONE', #3159, #3328, #116 ) ;
ENDSEC;
END-ISO-10303-21;
